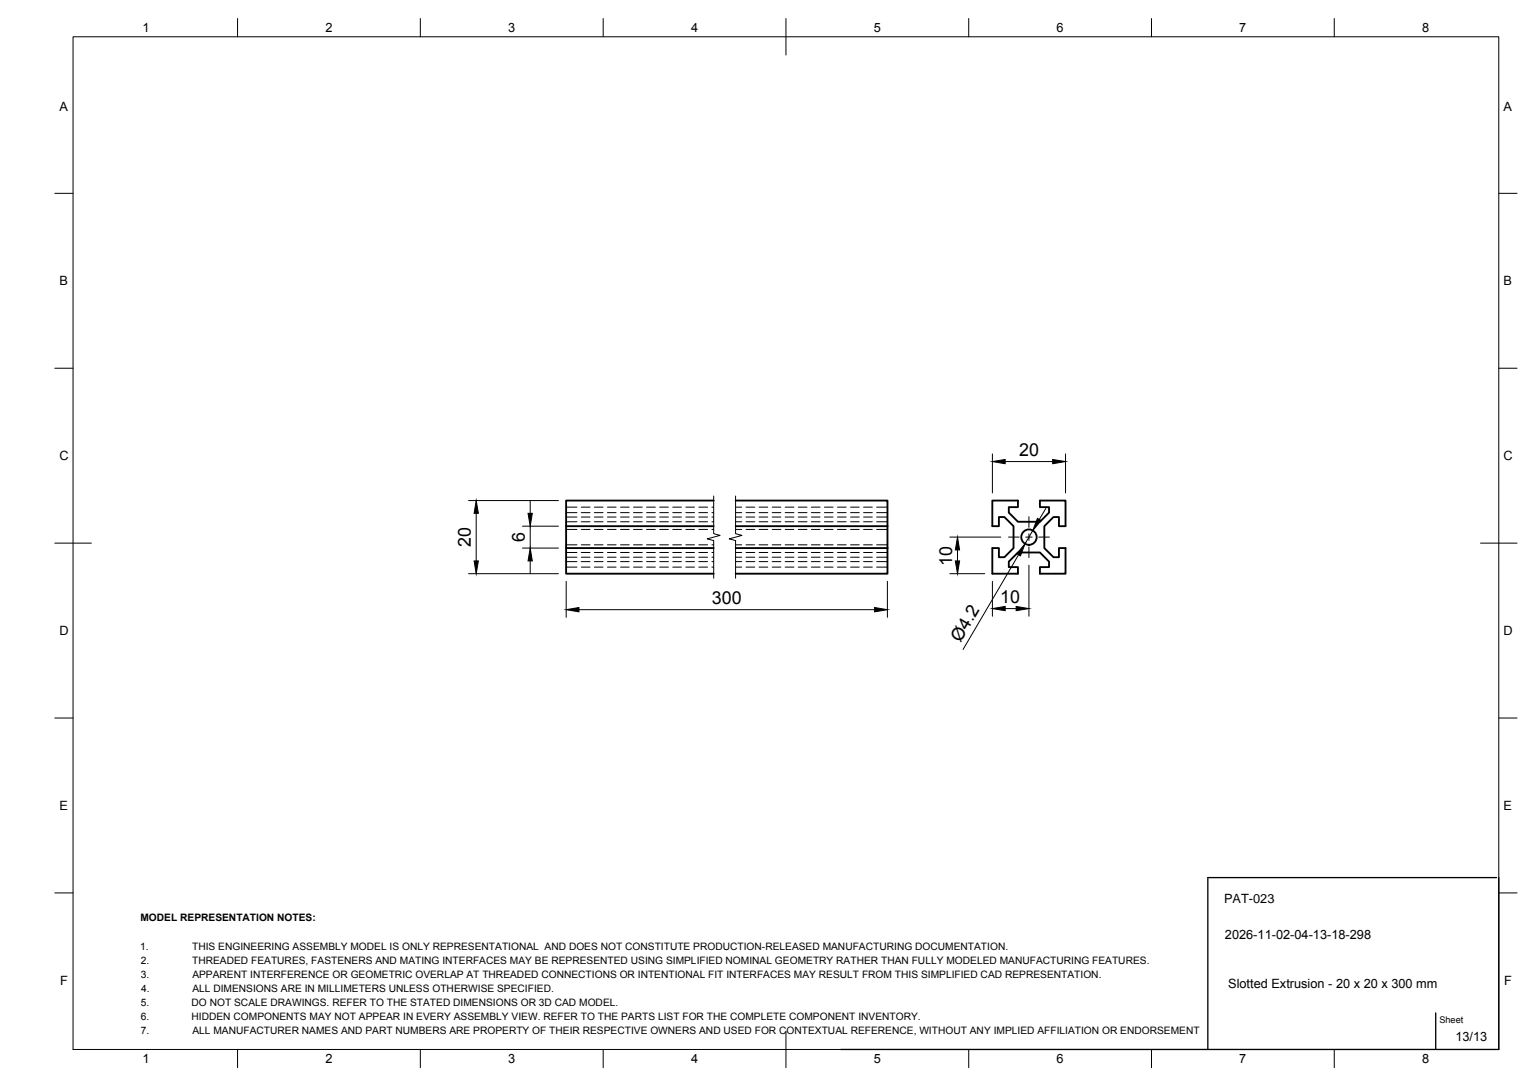
ISO-10303-21;
HEADER;
/* Generated by software containing ST-Developer
 * from STEP Tools, Inc. (www.steptools.com) 
 */

FILE_DESCRIPTION(
/* description */ ('PAT-023'),
/* implementation_level */ '2;1');

FILE_NAME(
/* name */ 'Slotted Extrusion - 20 x 20 x 300 mm.step',
/* time_stamp */ '2026-10-29T15:47:46-07:00',
/* author */ (''),
/* organization */ (''),
/* preprocessor_version */ 'ST-DEVELOPER v20.2',
/* originating_system */ 'Autodesk Translation Framework v15.17.0.0',
/* authorisation */ '');

FILE_SCHEMA (('AUTOMOTIVE_DESIGN { 1 0 10303 214 3 1 1 }'));
ENDSEC;

DATA;
#10=MECHANICAL_DESIGN_GEOMETRIC_PRESENTATION_REPRESENTATION('',(#91),#3773);
#75=SHAPE_REPRESENTATION_RELATIONSHIP('SRR','None',#3824,#83);
#83=ADVANCED_BREP_SHAPE_REPRESENTATION('',(#99),#3772);
#91=STYLED_ITEM('',(#3960),#99);
#99=MANIFOLD_SOLID_BREP('Body1',#2244);
#113=FACE_BOUND('',#468,.T.);
#114=FACE_BOUND('',#470,.T.);
#172=PLANE('',#2450);
#173=PLANE('',#2451);
#174=PLANE('',#2452);
#175=PLANE('',#2453);
#176=PLANE('',#2454);
#177=PLANE('',#2455);
#178=PLANE('',#2456);
#179=PLANE('',#2457);
#180=PLANE('',#2458);
#181=PLANE('',#2459);
#182=PLANE('',#2460);
#183=PLANE('',#2461);
#184=PLANE('',#2462);
#185=PLANE('',#2463);
#186=PLANE('',#2464);
#187=PLANE('',#2465);
#188=PLANE('',#2466);
#189=PLANE('',#2467);
#190=PLANE('',#2468);
#191=PLANE('',#2469);
#192=PLANE('',#2470);
#193=PLANE('',#2471);
#194=PLANE('',#2472);
#195=PLANE('',#2473);
#196=PLANE('',#2474);
#197=PLANE('',#2475);
#198=PLANE('',#2476);
#199=PLANE('',#2477);
#200=PLANE('',#2478);
#201=PLANE('',#2479);
#202=PLANE('',#2480);
#203=PLANE('',#2481);
#204=PLANE('',#2482);
#205=PLANE('',#2483);
#206=PLANE('',#2484);
#207=PLANE('',#2485);
#208=PLANE('',#2489);
#209=PLANE('',#2490);
#210=PLANE('',#2491);
#211=PLANE('',#2492);
#212=PLANE('',#2493);
#213=PLANE('',#2494);
#214=PLANE('',#2495);
#215=PLANE('',#2496);
#216=PLANE('',#2497);
#217=PLANE('',#2498);
#290=FACE_OUTER_BOUND('',#422,.T.);
#291=FACE_OUTER_BOUND('',#423,.T.);
#292=FACE_OUTER_BOUND('',#424,.T.);
#293=FACE_OUTER_BOUND('',#425,.T.);
#294=FACE_OUTER_BOUND('',#426,.T.);
#295=FACE_OUTER_BOUND('',#427,.T.);
#296=FACE_OUTER_BOUND('',#428,.T.);
#297=FACE_OUTER_BOUND('',#429,.T.);
#298=FACE_OUTER_BOUND('',#430,.T.);
#299=FACE_OUTER_BOUND('',#431,.T.);
#300=FACE_OUTER_BOUND('',#432,.T.);
#301=FACE_OUTER_BOUND('',#433,.T.);
#302=FACE_OUTER_BOUND('',#434,.T.);
#303=FACE_OUTER_BOUND('',#435,.T.);
#304=FACE_OUTER_BOUND('',#436,.T.);
#305=FACE_OUTER_BOUND('',#437,.T.);
#306=FACE_OUTER_BOUND('',#438,.T.);
#307=FACE_OUTER_BOUND('',#439,.T.);
#308=FACE_OUTER_BOUND('',#440,.T.);
#309=FACE_OUTER_BOUND('',#441,.T.);
#310=FACE_OUTER_BOUND('',#442,.T.);
#311=FACE_OUTER_BOUND('',#443,.T.);
#312=FACE_OUTER_BOUND('',#444,.T.);
#313=FACE_OUTER_BOUND('',#445,.T.);
#314=FACE_OUTER_BOUND('',#446,.T.);
#315=FACE_OUTER_BOUND('',#447,.T.);
#316=FACE_OUTER_BOUND('',#448,.T.);
#317=FACE_OUTER_BOUND('',#449,.T.);
#318=FACE_OUTER_BOUND('',#450,.T.);
#319=FACE_OUTER_BOUND('',#451,.T.);
#320=FACE_OUTER_BOUND('',#452,.T.);
#321=FACE_OUTER_BOUND('',#453,.T.);
#322=FACE_OUTER_BOUND('',#454,.T.);
#323=FACE_OUTER_BOUND('',#455,.T.);
#324=FACE_OUTER_BOUND('',#456,.T.);
#325=FACE_OUTER_BOUND('',#457,.T.);
#326=FACE_OUTER_BOUND('',#458,.T.);
#327=FACE_OUTER_BOUND('',#459,.T.);
#328=FACE_OUTER_BOUND('',#460,.T.);
#329=FACE_OUTER_BOUND('',#461,.T.);
#330=FACE_OUTER_BOUND('',#462,.T.);
#331=FACE_OUTER_BOUND('',#463,.T.);
#332=FACE_OUTER_BOUND('',#464,.T.);
#333=FACE_OUTER_BOUND('',#465,.T.);
#334=FACE_OUTER_BOUND('',#466,.T.);
#335=FACE_OUTER_BOUND('',#467,.T.);
#336=FACE_OUTER_BOUND('',#469,.T.);
#422=EDGE_LOOP('',(#1839,#1840,#1841,#1842));
#423=EDGE_LOOP('',(#1843,#1844,#1845,#1846));
#424=EDGE_LOOP('',(#1847,#1848,#1849,#1850));
#425=EDGE_LOOP('',(#1851,#1852,#1853,#1854));
#426=EDGE_LOOP('',(#1855,#1856,#1857,#1858));
#427=EDGE_LOOP('',(#1859,#1860,#1861,#1862));
#428=EDGE_LOOP('',(#1863,#1864,#1865,#1866));
#429=EDGE_LOOP('',(#1867,#1868,#1869,#1870));
#430=EDGE_LOOP('',(#1871,#1872,#1873,#1874));
#431=EDGE_LOOP('',(#1875,#1876,#1877,#1878));
#432=EDGE_LOOP('',(#1879,#1880,#1881,#1882));
#433=EDGE_LOOP('',(#1883,#1884,#1885,#1886));
#434=EDGE_LOOP('',(#1887,#1888,#1889,#1890));
#435=EDGE_LOOP('',(#1891,#1892,#1893,#1894));
#436=EDGE_LOOP('',(#1895,#1896,#1897,#1898));
#437=EDGE_LOOP('',(#1899,#1900,#1901,#1902));
#438=EDGE_LOOP('',(#1903,#1904,#1905,#1906));
#439=EDGE_LOOP('',(#1907,#1908,#1909,#1910));
#440=EDGE_LOOP('',(#1911,#1912,#1913,#1914));
#441=EDGE_LOOP('',(#1915,#1916,#1917,#1918));
#442=EDGE_LOOP('',(#1919,#1920,#1921,#1922));
#443=EDGE_LOOP('',(#1923,#1924,#1925,#1926));
#444=EDGE_LOOP('',(#1927,#1928,#1929,#1930));
#445=EDGE_LOOP('',(#1931,#1932,#1933,#1934));
#446=EDGE_LOOP('',(#1935,#1936,#1937,#1938));
#447=EDGE_LOOP('',(#1939,#1940,#1941,#1942));
#448=EDGE_LOOP('',(#1943,#1944,#1945,#1946));
#449=EDGE_LOOP('',(#1947,#1948,#1949,#1950));
#450=EDGE_LOOP('',(#1951,#1952,#1953,#1954));
#451=EDGE_LOOP('',(#1955,#1956,#1957,#1958));
#452=EDGE_LOOP('',(#1959,#1960,#1961,#1962));
#453=EDGE_LOOP('',(#1963,#1964,#1965,#1966));
#454=EDGE_LOOP('',(#1967,#1968,#1969,#1970));
#455=EDGE_LOOP('',(#1971,#1972,#1973,#1974));
#456=EDGE_LOOP('',(#1975,#1976,#1977,#1978));
#457=EDGE_LOOP('',(#1979,#1980,#1981,#1982));
#458=EDGE_LOOP('',(#1983,#1984,#1985,#1986));
#459=EDGE_LOOP('',(#1987,#1988,#1989,#1990));
#460=EDGE_LOOP('',(#1991,#1992,#1993,#1994));
#461=EDGE_LOOP('',(#1995,#1996,#1997,#1998));
#462=EDGE_LOOP('',(#1999,#2000,#2001,#2002));
#463=EDGE_LOOP('',(#2003,#2004,#2005,#2006));
#464=EDGE_LOOP('',(#2007,#2008,#2009,#2010));
#465=EDGE_LOOP('',(#2011,#2012,#2013,#2014));
#466=EDGE_LOOP('',(#2015,#2016,#2017,#2018));
#467=EDGE_LOOP('',(#2019,#2020,#2021,#2022,#2023,#2024,#2025,#2026,#2027,
#2028,#2029,#2030,#2031,#2032,#2033,#2034,#2035,#2036,#2037,#2038,#2039,
#2040,#2041,#2042,#2043,#2044,#2045,#2046,#2047,#2048,#2049,#2050,#2051,
#2052,#2053,#2054,#2055,#2056,#2057,#2058,#2059,#2060,#2061,#2062));
#468=EDGE_LOOP('',(#2063));
#469=EDGE_LOOP('',(#2064,#2065,#2066,#2067,#2068,#2069,#2070,#2071,#2072,
#2073,#2074,#2075,#2076,#2077,#2078,#2079,#2080,#2081,#2082,#2083,#2084,
#2085,#2086,#2087,#2088,#2089,#2090,#2091,#2092,#2093,#2094,#2095,#2096,
#2097,#2098,#2099,#2100,#2101,#2102,#2103,#2104,#2105,#2106,#2107));
#470=EDGE_LOOP('',(#2108));
#602=LINE('',#3476,#866);
#603=LINE('',#3478,#867);
#604=LINE('',#3480,#868);
#605=LINE('',#3481,#869);
#606=LINE('',#3484,#870);
#607=LINE('',#3486,#871);
#608=LINE('',#3487,#872);
#609=LINE('',#3490,#873);
#610=LINE('',#3492,#874);
#611=LINE('',#3493,#875);
#612=LINE('',#3496,#876);
#613=LINE('',#3498,#877);
#614=LINE('',#3499,#878);
#615=LINE('',#3502,#879);
#616=LINE('',#3504,#880);
#617=LINE('',#3505,#881);
#618=LINE('',#3508,#882);
#619=LINE('',#3510,#883);
#620=LINE('',#3511,#884);
#621=LINE('',#3514,#885);
#622=LINE('',#3516,#886);
#623=LINE('',#3517,#887);
#624=LINE('',#3520,#888);
#625=LINE('',#3522,#889);
#626=LINE('',#3523,#890);
#627=LINE('',#3526,#891);
#628=LINE('',#3528,#892);
#629=LINE('',#3529,#893);
#630=LINE('',#3533,#894);
#631=LINE('',#3535,#895);
#632=LINE('',#3537,#896);
#633=LINE('',#3538,#897);
#634=LINE('',#3541,#898);
#635=LINE('',#3543,#899);
#636=LINE('',#3544,#900);
#637=LINE('',#3547,#901);
#638=LINE('',#3549,#902);
#639=LINE('',#3550,#903);
#640=LINE('',#3553,#904);
#641=LINE('',#3555,#905);
#642=LINE('',#3556,#906);
#643=LINE('',#3559,#907);
#644=LINE('',#3561,#908);
#645=LINE('',#3562,#909);
#646=LINE('',#3565,#910);
#647=LINE('',#3567,#911);
#648=LINE('',#3568,#912);
#649=LINE('',#3571,#913);
#650=LINE('',#3573,#914);
#651=LINE('',#3574,#915);
#652=LINE('',#3577,#916);
#653=LINE('',#3579,#917);
#654=LINE('',#3580,#918);
#655=LINE('',#3583,#919);
#656=LINE('',#3585,#920);
#657=LINE('',#3586,#921);
#658=LINE('',#3590,#922);
#659=LINE('',#3592,#923);
#660=LINE('',#3594,#924);
#661=LINE('',#3595,#925);
#662=LINE('',#3598,#926);
#663=LINE('',#3600,#927);
#664=LINE('',#3601,#928);
#665=LINE('',#3604,#929);
#666=LINE('',#3606,#930);
#667=LINE('',#3607,#931);
#668=LINE('',#3610,#932);
#669=LINE('',#3612,#933);
#670=LINE('',#3613,#934);
#671=LINE('',#3616,#935);
#672=LINE('',#3618,#936);
#673=LINE('',#3619,#937);
#674=LINE('',#3622,#938);
#675=LINE('',#3624,#939);
#676=LINE('',#3625,#940);
#677=LINE('',#3628,#941);
#678=LINE('',#3630,#942);
#679=LINE('',#3631,#943);
#680=LINE('',#3634,#944);
#681=LINE('',#3636,#945);
#682=LINE('',#3637,#946);
#683=LINE('',#3640,#947);
#684=LINE('',#3642,#948);
#685=LINE('',#3643,#949);
#686=LINE('',#3647,#950);
#687=LINE('',#3649,#951);
#688=LINE('',#3651,#952);
#689=LINE('',#3652,#953);
#690=LINE('',#3655,#954);
#691=LINE('',#3657,#955);
#692=LINE('',#3658,#956);
#693=LINE('',#3661,#957);
#694=LINE('',#3663,#958);
#695=LINE('',#3664,#959);
#696=LINE('',#3667,#960);
#697=LINE('',#3669,#961);
#698=LINE('',#3670,#962);
#699=LINE('',#3673,#963);
#700=LINE('',#3675,#964);
#701=LINE('',#3676,#965);
#702=LINE('',#3679,#966);
#703=LINE('',#3681,#967);
#704=LINE('',#3682,#968);
#705=LINE('',#3685,#969);
#706=LINE('',#3687,#970);
#707=LINE('',#3688,#971);
#708=LINE('',#3691,#972);
#709=LINE('',#3693,#973);
#710=LINE('',#3694,#974);
#711=LINE('',#3697,#975);
#712=LINE('',#3699,#976);
#713=LINE('',#3700,#977);
#714=LINE('',#3705,#978);
#715=LINE('',#3709,#979);
#716=LINE('',#3711,#980);
#717=LINE('',#3712,#981);
#718=LINE('',#3715,#982);
#719=LINE('',#3717,#983);
#720=LINE('',#3718,#984);
#721=LINE('',#3720,#985);
#722=LINE('',#3721,#986);
#723=LINE('',#3724,#987);
#724=LINE('',#3726,#988);
#725=LINE('',#3727,#989);
#726=LINE('',#3729,#990);
#727=LINE('',#3730,#991);
#728=LINE('',#3733,#992);
#729=LINE('',#3735,#993);
#730=LINE('',#3736,#994);
#731=LINE('',#3738,#995);
#732=LINE('',#3739,#996);
#733=LINE('',#3741,#997);
#734=LINE('',#3742,#998);
#866=VECTOR('',#2867,1.);
#867=VECTOR('',#2868,1.);
#868=VECTOR('',#2869,1.);
#869=VECTOR('',#2870,1.);
#870=VECTOR('',#2873,1.);
#871=VECTOR('',#2874,1.);
#872=VECTOR('',#2875,1.);
#873=VECTOR('',#2878,1.);
#874=VECTOR('',#2879,1.);
#875=VECTOR('',#2880,1.);
#876=VECTOR('',#2883,1.);
#877=VECTOR('',#2884,1.);
#878=VECTOR('',#2885,1.);
#879=VECTOR('',#2888,1.);
#880=VECTOR('',#2889,1.);
#881=VECTOR('',#2890,1.);
#882=VECTOR('',#2893,1.);
#883=VECTOR('',#2894,1.);
#884=VECTOR('',#2895,1.);
#885=VECTOR('',#2898,1.);
#886=VECTOR('',#2899,1.);
#887=VECTOR('',#2900,1.);
#888=VECTOR('',#2903,1.);
#889=VECTOR('',#2904,1.);
#890=VECTOR('',#2905,1.);
#891=VECTOR('',#2908,1.);
#892=VECTOR('',#2909,1.);
#893=VECTOR('',#2910,1.);
#894=VECTOR('',#2913,1.);
#895=VECTOR('',#2914,1.);
#896=VECTOR('',#2915,1.);
#897=VECTOR('',#2916,1.);
#898=VECTOR('',#2919,1.);
#899=VECTOR('',#2920,1.);
#900=VECTOR('',#2921,1.);
#901=VECTOR('',#2924,1.);
#902=VECTOR('',#2925,1.);
#903=VECTOR('',#2926,1.);
#904=VECTOR('',#2929,1.);
#905=VECTOR('',#2930,1.);
#906=VECTOR('',#2931,1.);
#907=VECTOR('',#2934,1.);
#908=VECTOR('',#2935,1.);
#909=VECTOR('',#2936,1.);
#910=VECTOR('',#2939,1.);
#911=VECTOR('',#2940,1.);
#912=VECTOR('',#2941,1.);
#913=VECTOR('',#2944,1.);
#914=VECTOR('',#2945,1.);
#915=VECTOR('',#2946,1.);
#916=VECTOR('',#2949,1.);
#917=VECTOR('',#2950,1.);
#918=VECTOR('',#2951,1.);
#919=VECTOR('',#2954,1.);
#920=VECTOR('',#2955,1.);
#921=VECTOR('',#2956,1.);
#922=VECTOR('',#2959,1.);
#923=VECTOR('',#2960,1.);
#924=VECTOR('',#2961,1.);
#925=VECTOR('',#2962,1.);
#926=VECTOR('',#2965,1.);
#927=VECTOR('',#2966,1.);
#928=VECTOR('',#2967,1.);
#929=VECTOR('',#2970,1.);
#930=VECTOR('',#2971,1.);
#931=VECTOR('',#2972,1.);
#932=VECTOR('',#2975,1.);
#933=VECTOR('',#2976,1.);
#934=VECTOR('',#2977,1.);
#935=VECTOR('',#2980,1.);
#936=VECTOR('',#2981,1.);
#937=VECTOR('',#2982,1.);
#938=VECTOR('',#2985,1.);
#939=VECTOR('',#2986,1.);
#940=VECTOR('',#2987,1.);
#941=VECTOR('',#2990,1.);
#942=VECTOR('',#2991,1.);
#943=VECTOR('',#2992,1.);
#944=VECTOR('',#2995,1.);
#945=VECTOR('',#2996,1.);
#946=VECTOR('',#2997,1.);
#947=VECTOR('',#3000,1.);
#948=VECTOR('',#3001,1.);
#949=VECTOR('',#3002,1.);
#950=VECTOR('',#3005,1.);
#951=VECTOR('',#3006,1.);
#952=VECTOR('',#3007,1.);
#953=VECTOR('',#3008,1.);
#954=VECTOR('',#3011,1.);
#955=VECTOR('',#3012,1.);
#956=VECTOR('',#3013,1.);
#957=VECTOR('',#3016,1.);
#958=VECTOR('',#3017,1.);
#959=VECTOR('',#3018,1.);
#960=VECTOR('',#3021,1.);
#961=VECTOR('',#3022,1.);
#962=VECTOR('',#3023,1.);
#963=VECTOR('',#3026,1.);
#964=VECTOR('',#3027,1.);
#965=VECTOR('',#3028,1.);
#966=VECTOR('',#3031,1.);
#967=VECTOR('',#3032,1.);
#968=VECTOR('',#3033,1.);
#969=VECTOR('',#3036,1.);
#970=VECTOR('',#3037,1.);
#971=VECTOR('',#3038,1.);
#972=VECTOR('',#3041,1.);
#973=VECTOR('',#3042,1.);
#974=VECTOR('',#3043,1.);
#975=VECTOR('',#3046,1.);
#976=VECTOR('',#3047,1.);
#977=VECTOR('',#3048,1.);
#978=VECTOR('',#3053,0.21);
#979=VECTOR('',#3058,1.);
#980=VECTOR('',#3059,1.);
#981=VECTOR('',#3060,1.);
#982=VECTOR('',#3063,1.);
#983=VECTOR('',#3064,1.);
#984=VECTOR('',#3065,1.);
#985=VECTOR('',#3068,1.);
#986=VECTOR('',#3069,1.);
#987=VECTOR('',#3072,1.);
#988=VECTOR('',#3073,1.);
#989=VECTOR('',#3074,1.);
#990=VECTOR('',#3077,1.);
#991=VECTOR('',#3078,1.);
#992=VECTOR('',#3081,1.);
#993=VECTOR('',#3082,1.);
#994=VECTOR('',#3083,1.);
#995=VECTOR('',#3086,1.);
#996=VECTOR('',#3087,1.);
#997=VECTOR('',#3090,1.);
#998=VECTOR('',#3091,1.);
#1023=CIRCLE('',#2487,0.21);
#1024=CIRCLE('',#2488,0.21);
#1131=VERTEX_POINT('',#3474);
#1132=VERTEX_POINT('',#3475);
#1133=VERTEX_POINT('',#3477);
#1134=VERTEX_POINT('',#3479);
#1135=VERTEX_POINT('',#3483);
#1136=VERTEX_POINT('',#3485);
#1137=VERTEX_POINT('',#3489);
#1138=VERTEX_POINT('',#3491);
#1139=VERTEX_POINT('',#3495);
#1140=VERTEX_POINT('',#3497);
#1141=VERTEX_POINT('',#3501);
#1142=VERTEX_POINT('',#3503);
#1143=VERTEX_POINT('',#3507);
#1144=VERTEX_POINT('',#3509);
#1145=VERTEX_POINT('',#3513);
#1146=VERTEX_POINT('',#3515);
#1147=VERTEX_POINT('',#3519);
#1148=VERTEX_POINT('',#3521);
#1149=VERTEX_POINT('',#3525);
#1150=VERTEX_POINT('',#3527);
#1151=VERTEX_POINT('',#3531);
#1152=VERTEX_POINT('',#3532);
#1153=VERTEX_POINT('',#3534);
#1154=VERTEX_POINT('',#3536);
#1155=VERTEX_POINT('',#3540);
#1156=VERTEX_POINT('',#3542);
#1157=VERTEX_POINT('',#3546);
#1158=VERTEX_POINT('',#3548);
#1159=VERTEX_POINT('',#3552);
#1160=VERTEX_POINT('',#3554);
#1161=VERTEX_POINT('',#3558);
#1162=VERTEX_POINT('',#3560);
#1163=VERTEX_POINT('',#3564);
#1164=VERTEX_POINT('',#3566);
#1165=VERTEX_POINT('',#3570);
#1166=VERTEX_POINT('',#3572);
#1167=VERTEX_POINT('',#3576);
#1168=VERTEX_POINT('',#3578);
#1169=VERTEX_POINT('',#3582);
#1170=VERTEX_POINT('',#3584);
#1171=VERTEX_POINT('',#3588);
#1172=VERTEX_POINT('',#3589);
#1173=VERTEX_POINT('',#3591);
#1174=VERTEX_POINT('',#3593);
#1175=VERTEX_POINT('',#3597);
#1176=VERTEX_POINT('',#3599);
#1177=VERTEX_POINT('',#3603);
#1178=VERTEX_POINT('',#3605);
#1179=VERTEX_POINT('',#3609);
#1180=VERTEX_POINT('',#3611);
#1181=VERTEX_POINT('',#3615);
#1182=VERTEX_POINT('',#3617);
#1183=VERTEX_POINT('',#3621);
#1184=VERTEX_POINT('',#3623);
#1185=VERTEX_POINT('',#3627);
#1186=VERTEX_POINT('',#3629);
#1187=VERTEX_POINT('',#3633);
#1188=VERTEX_POINT('',#3635);
#1189=VERTEX_POINT('',#3639);
#1190=VERTEX_POINT('',#3641);
#1191=VERTEX_POINT('',#3645);
#1192=VERTEX_POINT('',#3646);
#1193=VERTEX_POINT('',#3648);
#1194=VERTEX_POINT('',#3650);
#1195=VERTEX_POINT('',#3654);
#1196=VERTEX_POINT('',#3656);
#1197=VERTEX_POINT('',#3660);
#1198=VERTEX_POINT('',#3662);
#1199=VERTEX_POINT('',#3666);
#1200=VERTEX_POINT('',#3668);
#1201=VERTEX_POINT('',#3672);
#1202=VERTEX_POINT('',#3674);
#1203=VERTEX_POINT('',#3678);
#1204=VERTEX_POINT('',#3680);
#1205=VERTEX_POINT('',#3684);
#1206=VERTEX_POINT('',#3686);
#1207=VERTEX_POINT('',#3690);
#1208=VERTEX_POINT('',#3692);
#1209=VERTEX_POINT('',#3696);
#1210=VERTEX_POINT('',#3698);
#1211=VERTEX_POINT('',#3702);
#1212=VERTEX_POINT('',#3704);
#1213=VERTEX_POINT('',#3708);
#1214=VERTEX_POINT('',#3710);
#1215=VERTEX_POINT('',#3714);
#1216=VERTEX_POINT('',#3716);
#1217=VERTEX_POINT('',#3723);
#1218=VERTEX_POINT('',#3725);
#1219=VERTEX_POINT('',#3732);
#1220=VERTEX_POINT('',#3734);
#1382=EDGE_CURVE('',#1131,#1132,#602,.T.);
#1383=EDGE_CURVE('',#1131,#1133,#603,.T.);
#1384=EDGE_CURVE('',#1134,#1133,#604,.T.);
#1385=EDGE_CURVE('',#1132,#1134,#605,.T.);
#1386=EDGE_CURVE('',#1135,#1131,#606,.T.);
#1387=EDGE_CURVE('',#1135,#1136,#607,.T.);
#1388=EDGE_CURVE('',#1133,#1136,#608,.T.);
#1389=EDGE_CURVE('',#1137,#1135,#609,.T.);
#1390=EDGE_CURVE('',#1137,#1138,#610,.T.);
#1391=EDGE_CURVE('',#1136,#1138,#611,.T.);
#1392=EDGE_CURVE('',#1139,#1137,#612,.T.);
#1393=EDGE_CURVE('',#1139,#1140,#613,.T.);
#1394=EDGE_CURVE('',#1138,#1140,#614,.T.);
#1395=EDGE_CURVE('',#1141,#1139,#615,.T.);
#1396=EDGE_CURVE('',#1141,#1142,#616,.T.);
#1397=EDGE_CURVE('',#1140,#1142,#617,.T.);
#1398=EDGE_CURVE('',#1143,#1141,#618,.T.);
#1399=EDGE_CURVE('',#1143,#1144,#619,.T.);
#1400=EDGE_CURVE('',#1142,#1144,#620,.T.);
#1401=EDGE_CURVE('',#1145,#1143,#621,.T.);
#1402=EDGE_CURVE('',#1145,#1146,#622,.T.);
#1403=EDGE_CURVE('',#1144,#1146,#623,.T.);
#1404=EDGE_CURVE('',#1147,#1145,#624,.T.);
#1405=EDGE_CURVE('',#1147,#1148,#625,.T.);
#1406=EDGE_CURVE('',#1146,#1148,#626,.T.);
#1407=EDGE_CURVE('',#1149,#1147,#627,.T.);
#1408=EDGE_CURVE('',#1150,#1149,#628,.T.);
#1409=EDGE_CURVE('',#1148,#1150,#629,.T.);
#1410=EDGE_CURVE('',#1151,#1152,#630,.T.);
#1411=EDGE_CURVE('',#1151,#1153,#631,.T.);
#1412=EDGE_CURVE('',#1154,#1153,#632,.T.);
#1413=EDGE_CURVE('',#1152,#1154,#633,.T.);
#1414=EDGE_CURVE('',#1155,#1151,#634,.T.);
#1415=EDGE_CURVE('',#1155,#1156,#635,.T.);
#1416=EDGE_CURVE('',#1153,#1156,#636,.T.);
#1417=EDGE_CURVE('',#1157,#1155,#637,.T.);
#1418=EDGE_CURVE('',#1157,#1158,#638,.T.);
#1419=EDGE_CURVE('',#1156,#1158,#639,.T.);
#1420=EDGE_CURVE('',#1159,#1157,#640,.T.);
#1421=EDGE_CURVE('',#1159,#1160,#641,.T.);
#1422=EDGE_CURVE('',#1158,#1160,#642,.T.);
#1423=EDGE_CURVE('',#1161,#1159,#643,.T.);
#1424=EDGE_CURVE('',#1161,#1162,#644,.T.);
#1425=EDGE_CURVE('',#1160,#1162,#645,.T.);
#1426=EDGE_CURVE('',#1163,#1161,#646,.T.);
#1427=EDGE_CURVE('',#1163,#1164,#647,.T.);
#1428=EDGE_CURVE('',#1162,#1164,#648,.T.);
#1429=EDGE_CURVE('',#1165,#1163,#649,.T.);
#1430=EDGE_CURVE('',#1165,#1166,#650,.T.);
#1431=EDGE_CURVE('',#1164,#1166,#651,.T.);
#1432=EDGE_CURVE('',#1167,#1165,#652,.T.);
#1433=EDGE_CURVE('',#1167,#1168,#653,.T.);
#1434=EDGE_CURVE('',#1166,#1168,#654,.T.);
#1435=EDGE_CURVE('',#1169,#1167,#655,.T.);
#1436=EDGE_CURVE('',#1170,#1169,#656,.T.);
#1437=EDGE_CURVE('',#1168,#1170,#657,.T.);
#1438=EDGE_CURVE('',#1171,#1172,#658,.T.);
#1439=EDGE_CURVE('',#1171,#1173,#659,.T.);
#1440=EDGE_CURVE('',#1174,#1173,#660,.T.);
#1441=EDGE_CURVE('',#1172,#1174,#661,.T.);
#1442=EDGE_CURVE('',#1175,#1171,#662,.T.);
#1443=EDGE_CURVE('',#1175,#1176,#663,.T.);
#1444=EDGE_CURVE('',#1173,#1176,#664,.T.);
#1445=EDGE_CURVE('',#1177,#1175,#665,.T.);
#1446=EDGE_CURVE('',#1177,#1178,#666,.T.);
#1447=EDGE_CURVE('',#1176,#1178,#667,.T.);
#1448=EDGE_CURVE('',#1179,#1177,#668,.T.);
#1449=EDGE_CURVE('',#1179,#1180,#669,.T.);
#1450=EDGE_CURVE('',#1178,#1180,#670,.T.);
#1451=EDGE_CURVE('',#1181,#1179,#671,.T.);
#1452=EDGE_CURVE('',#1181,#1182,#672,.T.);
#1453=EDGE_CURVE('',#1180,#1182,#673,.T.);
#1454=EDGE_CURVE('',#1183,#1181,#674,.T.);
#1455=EDGE_CURVE('',#1183,#1184,#675,.T.);
#1456=EDGE_CURVE('',#1182,#1184,#676,.T.);
#1457=EDGE_CURVE('',#1185,#1183,#677,.T.);
#1458=EDGE_CURVE('',#1185,#1186,#678,.T.);
#1459=EDGE_CURVE('',#1184,#1186,#679,.T.);
#1460=EDGE_CURVE('',#1187,#1185,#680,.T.);
#1461=EDGE_CURVE('',#1187,#1188,#681,.T.);
#1462=EDGE_CURVE('',#1186,#1188,#682,.T.);
#1463=EDGE_CURVE('',#1189,#1187,#683,.T.);
#1464=EDGE_CURVE('',#1190,#1189,#684,.T.);
#1465=EDGE_CURVE('',#1188,#1190,#685,.T.);
#1466=EDGE_CURVE('',#1191,#1192,#686,.T.);
#1467=EDGE_CURVE('',#1191,#1193,#687,.T.);
#1468=EDGE_CURVE('',#1194,#1193,#688,.T.);
#1469=EDGE_CURVE('',#1192,#1194,#689,.T.);
#1470=EDGE_CURVE('',#1195,#1191,#690,.T.);
#1471=EDGE_CURVE('',#1195,#1196,#691,.T.);
#1472=EDGE_CURVE('',#1193,#1196,#692,.T.);
#1473=EDGE_CURVE('',#1197,#1195,#693,.T.);
#1474=EDGE_CURVE('',#1197,#1198,#694,.T.);
#1475=EDGE_CURVE('',#1196,#1198,#695,.T.);
#1476=EDGE_CURVE('',#1199,#1197,#696,.T.);
#1477=EDGE_CURVE('',#1199,#1200,#697,.T.);
#1478=EDGE_CURVE('',#1198,#1200,#698,.T.);
#1479=EDGE_CURVE('',#1201,#1199,#699,.T.);
#1480=EDGE_CURVE('',#1201,#1202,#700,.T.);
#1481=EDGE_CURVE('',#1200,#1202,#701,.T.);
#1482=EDGE_CURVE('',#1203,#1201,#702,.T.);
#1483=EDGE_CURVE('',#1203,#1204,#703,.T.);
#1484=EDGE_CURVE('',#1202,#1204,#704,.T.);
#1485=EDGE_CURVE('',#1205,#1203,#705,.T.);
#1486=EDGE_CURVE('',#1205,#1206,#706,.T.);
#1487=EDGE_CURVE('',#1204,#1206,#707,.T.);
#1488=EDGE_CURVE('',#1207,#1205,#708,.T.);
#1489=EDGE_CURVE('',#1207,#1208,#709,.T.);
#1490=EDGE_CURVE('',#1206,#1208,#710,.T.);
#1491=EDGE_CURVE('',#1209,#1207,#711,.T.);
#1492=EDGE_CURVE('',#1210,#1209,#712,.T.);
#1493=EDGE_CURVE('',#1208,#1210,#713,.T.);
#1494=EDGE_CURVE('',#1211,#1211,#1023,.T.);
#1495=EDGE_CURVE('',#1211,#1212,#714,.T.);
#1496=EDGE_CURVE('',#1212,#1212,#1024,.T.);
#1497=EDGE_CURVE('',#1149,#1213,#715,.T.);
#1498=EDGE_CURVE('',#1213,#1214,#716,.T.);
#1499=EDGE_CURVE('',#1150,#1214,#717,.T.);
#1500=EDGE_CURVE('',#1215,#1134,#718,.T.);
#1501=EDGE_CURVE('',#1216,#1215,#719,.T.);
#1502=EDGE_CURVE('',#1216,#1132,#720,.T.);
#1503=EDGE_CURVE('',#1169,#1216,#721,.T.);
#1504=EDGE_CURVE('',#1170,#1215,#722,.T.);
#1505=EDGE_CURVE('',#1217,#1154,#723,.T.);
#1506=EDGE_CURVE('',#1218,#1217,#724,.T.);
#1507=EDGE_CURVE('',#1218,#1152,#725,.T.);
#1508=EDGE_CURVE('',#1189,#1218,#726,.T.);
#1509=EDGE_CURVE('',#1190,#1217,#727,.T.);
#1510=EDGE_CURVE('',#1219,#1174,#728,.T.);
#1511=EDGE_CURVE('',#1220,#1219,#729,.T.);
#1512=EDGE_CURVE('',#1220,#1172,#730,.T.);
#1513=EDGE_CURVE('',#1209,#1220,#731,.T.);
#1514=EDGE_CURVE('',#1210,#1219,#732,.T.);
#1515=EDGE_CURVE('',#1214,#1194,#733,.T.);
#1516=EDGE_CURVE('',#1213,#1192,#734,.T.);
#1839=ORIENTED_EDGE('',*,*,#1382,.F.);
#1840=ORIENTED_EDGE('',*,*,#1383,.T.);
#1841=ORIENTED_EDGE('',*,*,#1384,.F.);
#1842=ORIENTED_EDGE('',*,*,#1385,.F.);
#1843=ORIENTED_EDGE('',*,*,#1386,.F.);
#1844=ORIENTED_EDGE('',*,*,#1387,.T.);
#1845=ORIENTED_EDGE('',*,*,#1388,.F.);
#1846=ORIENTED_EDGE('',*,*,#1383,.F.);
#1847=ORIENTED_EDGE('',*,*,#1389,.F.);
#1848=ORIENTED_EDGE('',*,*,#1390,.T.);
#1849=ORIENTED_EDGE('',*,*,#1391,.F.);
#1850=ORIENTED_EDGE('',*,*,#1387,.F.);
#1851=ORIENTED_EDGE('',*,*,#1392,.F.);
#1852=ORIENTED_EDGE('',*,*,#1393,.T.);
#1853=ORIENTED_EDGE('',*,*,#1394,.F.);
#1854=ORIENTED_EDGE('',*,*,#1390,.F.);
#1855=ORIENTED_EDGE('',*,*,#1395,.F.);
#1856=ORIENTED_EDGE('',*,*,#1396,.T.);
#1857=ORIENTED_EDGE('',*,*,#1397,.F.);
#1858=ORIENTED_EDGE('',*,*,#1393,.F.);
#1859=ORIENTED_EDGE('',*,*,#1398,.F.);
#1860=ORIENTED_EDGE('',*,*,#1399,.T.);
#1861=ORIENTED_EDGE('',*,*,#1400,.F.);
#1862=ORIENTED_EDGE('',*,*,#1396,.F.);
#1863=ORIENTED_EDGE('',*,*,#1401,.F.);
#1864=ORIENTED_EDGE('',*,*,#1402,.T.);
#1865=ORIENTED_EDGE('',*,*,#1403,.F.);
#1866=ORIENTED_EDGE('',*,*,#1399,.F.);
#1867=ORIENTED_EDGE('',*,*,#1404,.F.);
#1868=ORIENTED_EDGE('',*,*,#1405,.T.);
#1869=ORIENTED_EDGE('',*,*,#1406,.F.);
#1870=ORIENTED_EDGE('',*,*,#1402,.F.);
#1871=ORIENTED_EDGE('',*,*,#1407,.F.);
#1872=ORIENTED_EDGE('',*,*,#1408,.F.);
#1873=ORIENTED_EDGE('',*,*,#1409,.F.);
#1874=ORIENTED_EDGE('',*,*,#1405,.F.);
#1875=ORIENTED_EDGE('',*,*,#1410,.F.);
#1876=ORIENTED_EDGE('',*,*,#1411,.T.);
#1877=ORIENTED_EDGE('',*,*,#1412,.F.);
#1878=ORIENTED_EDGE('',*,*,#1413,.F.);
#1879=ORIENTED_EDGE('',*,*,#1414,.F.);
#1880=ORIENTED_EDGE('',*,*,#1415,.T.);
#1881=ORIENTED_EDGE('',*,*,#1416,.F.);
#1882=ORIENTED_EDGE('',*,*,#1411,.F.);
#1883=ORIENTED_EDGE('',*,*,#1417,.F.);
#1884=ORIENTED_EDGE('',*,*,#1418,.T.);
#1885=ORIENTED_EDGE('',*,*,#1419,.F.);
#1886=ORIENTED_EDGE('',*,*,#1415,.F.);
#1887=ORIENTED_EDGE('',*,*,#1420,.F.);
#1888=ORIENTED_EDGE('',*,*,#1421,.T.);
#1889=ORIENTED_EDGE('',*,*,#1422,.F.);
#1890=ORIENTED_EDGE('',*,*,#1418,.F.);
#1891=ORIENTED_EDGE('',*,*,#1423,.F.);
#1892=ORIENTED_EDGE('',*,*,#1424,.T.);
#1893=ORIENTED_EDGE('',*,*,#1425,.F.);
#1894=ORIENTED_EDGE('',*,*,#1421,.F.);
#1895=ORIENTED_EDGE('',*,*,#1426,.F.);
#1896=ORIENTED_EDGE('',*,*,#1427,.T.);
#1897=ORIENTED_EDGE('',*,*,#1428,.F.);
#1898=ORIENTED_EDGE('',*,*,#1424,.F.);
#1899=ORIENTED_EDGE('',*,*,#1429,.F.);
#1900=ORIENTED_EDGE('',*,*,#1430,.T.);
#1901=ORIENTED_EDGE('',*,*,#1431,.F.);
#1902=ORIENTED_EDGE('',*,*,#1427,.F.);
#1903=ORIENTED_EDGE('',*,*,#1432,.F.);
#1904=ORIENTED_EDGE('',*,*,#1433,.T.);
#1905=ORIENTED_EDGE('',*,*,#1434,.F.);
#1906=ORIENTED_EDGE('',*,*,#1430,.F.);
#1907=ORIENTED_EDGE('',*,*,#1435,.F.);
#1908=ORIENTED_EDGE('',*,*,#1436,.F.);
#1909=ORIENTED_EDGE('',*,*,#1437,.F.);
#1910=ORIENTED_EDGE('',*,*,#1433,.F.);
#1911=ORIENTED_EDGE('',*,*,#1438,.F.);
#1912=ORIENTED_EDGE('',*,*,#1439,.T.);
#1913=ORIENTED_EDGE('',*,*,#1440,.F.);
#1914=ORIENTED_EDGE('',*,*,#1441,.F.);
#1915=ORIENTED_EDGE('',*,*,#1442,.F.);
#1916=ORIENTED_EDGE('',*,*,#1443,.T.);
#1917=ORIENTED_EDGE('',*,*,#1444,.F.);
#1918=ORIENTED_EDGE('',*,*,#1439,.F.);
#1919=ORIENTED_EDGE('',*,*,#1445,.F.);
#1920=ORIENTED_EDGE('',*,*,#1446,.T.);
#1921=ORIENTED_EDGE('',*,*,#1447,.F.);
#1922=ORIENTED_EDGE('',*,*,#1443,.F.);
#1923=ORIENTED_EDGE('',*,*,#1448,.F.);
#1924=ORIENTED_EDGE('',*,*,#1449,.T.);
#1925=ORIENTED_EDGE('',*,*,#1450,.F.);
#1926=ORIENTED_EDGE('',*,*,#1446,.F.);
#1927=ORIENTED_EDGE('',*,*,#1451,.F.);
#1928=ORIENTED_EDGE('',*,*,#1452,.T.);
#1929=ORIENTED_EDGE('',*,*,#1453,.F.);
#1930=ORIENTED_EDGE('',*,*,#1449,.F.);
#1931=ORIENTED_EDGE('',*,*,#1454,.F.);
#1932=ORIENTED_EDGE('',*,*,#1455,.T.);
#1933=ORIENTED_EDGE('',*,*,#1456,.F.);
#1934=ORIENTED_EDGE('',*,*,#1452,.F.);
#1935=ORIENTED_EDGE('',*,*,#1457,.F.);
#1936=ORIENTED_EDGE('',*,*,#1458,.T.);
#1937=ORIENTED_EDGE('',*,*,#1459,.F.);
#1938=ORIENTED_EDGE('',*,*,#1455,.F.);
#1939=ORIENTED_EDGE('',*,*,#1460,.F.);
#1940=ORIENTED_EDGE('',*,*,#1461,.T.);
#1941=ORIENTED_EDGE('',*,*,#1462,.F.);
#1942=ORIENTED_EDGE('',*,*,#1458,.F.);
#1943=ORIENTED_EDGE('',*,*,#1463,.F.);
#1944=ORIENTED_EDGE('',*,*,#1464,.F.);
#1945=ORIENTED_EDGE('',*,*,#1465,.F.);
#1946=ORIENTED_EDGE('',*,*,#1461,.F.);
#1947=ORIENTED_EDGE('',*,*,#1466,.F.);
#1948=ORIENTED_EDGE('',*,*,#1467,.T.);
#1949=ORIENTED_EDGE('',*,*,#1468,.F.);
#1950=ORIENTED_EDGE('',*,*,#1469,.F.);
#1951=ORIENTED_EDGE('',*,*,#1470,.F.);
#1952=ORIENTED_EDGE('',*,*,#1471,.T.);
#1953=ORIENTED_EDGE('',*,*,#1472,.F.);
#1954=ORIENTED_EDGE('',*,*,#1467,.F.);
#1955=ORIENTED_EDGE('',*,*,#1473,.F.);
#1956=ORIENTED_EDGE('',*,*,#1474,.T.);
#1957=ORIENTED_EDGE('',*,*,#1475,.F.);
#1958=ORIENTED_EDGE('',*,*,#1471,.F.);
#1959=ORIENTED_EDGE('',*,*,#1476,.F.);
#1960=ORIENTED_EDGE('',*,*,#1477,.T.);
#1961=ORIENTED_EDGE('',*,*,#1478,.F.);
#1962=ORIENTED_EDGE('',*,*,#1474,.F.);
#1963=ORIENTED_EDGE('',*,*,#1479,.F.);
#1964=ORIENTED_EDGE('',*,*,#1480,.T.);
#1965=ORIENTED_EDGE('',*,*,#1481,.F.);
#1966=ORIENTED_EDGE('',*,*,#1477,.F.);
#1967=ORIENTED_EDGE('',*,*,#1482,.F.);
#1968=ORIENTED_EDGE('',*,*,#1483,.T.);
#1969=ORIENTED_EDGE('',*,*,#1484,.F.);
#1970=ORIENTED_EDGE('',*,*,#1480,.F.);
#1971=ORIENTED_EDGE('',*,*,#1485,.F.);
#1972=ORIENTED_EDGE('',*,*,#1486,.T.);
#1973=ORIENTED_EDGE('',*,*,#1487,.F.);
#1974=ORIENTED_EDGE('',*,*,#1483,.F.);
#1975=ORIENTED_EDGE('',*,*,#1488,.F.);
#1976=ORIENTED_EDGE('',*,*,#1489,.T.);
#1977=ORIENTED_EDGE('',*,*,#1490,.F.);
#1978=ORIENTED_EDGE('',*,*,#1486,.F.);
#1979=ORIENTED_EDGE('',*,*,#1491,.F.);
#1980=ORIENTED_EDGE('',*,*,#1492,.F.);
#1981=ORIENTED_EDGE('',*,*,#1493,.F.);
#1982=ORIENTED_EDGE('',*,*,#1489,.F.);
#1983=ORIENTED_EDGE('',*,*,#1494,.F.);
#1984=ORIENTED_EDGE('',*,*,#1495,.T.);
#1985=ORIENTED_EDGE('',*,*,#1496,.F.);
#1986=ORIENTED_EDGE('',*,*,#1495,.F.);
#1987=ORIENTED_EDGE('',*,*,#1408,.T.);
#1988=ORIENTED_EDGE('',*,*,#1497,.T.);
#1989=ORIENTED_EDGE('',*,*,#1498,.T.);
#1990=ORIENTED_EDGE('',*,*,#1499,.F.);
#1991=ORIENTED_EDGE('',*,*,#1385,.T.);
#1992=ORIENTED_EDGE('',*,*,#1500,.F.);
#1993=ORIENTED_EDGE('',*,*,#1501,.F.);
#1994=ORIENTED_EDGE('',*,*,#1502,.T.);
#1995=ORIENTED_EDGE('',*,*,#1436,.T.);
#1996=ORIENTED_EDGE('',*,*,#1503,.T.);
#1997=ORIENTED_EDGE('',*,*,#1501,.T.);
#1998=ORIENTED_EDGE('',*,*,#1504,.F.);
#1999=ORIENTED_EDGE('',*,*,#1413,.T.);
#2000=ORIENTED_EDGE('',*,*,#1505,.F.);
#2001=ORIENTED_EDGE('',*,*,#1506,.F.);
#2002=ORIENTED_EDGE('',*,*,#1507,.T.);
#2003=ORIENTED_EDGE('',*,*,#1464,.T.);
#2004=ORIENTED_EDGE('',*,*,#1508,.T.);
#2005=ORIENTED_EDGE('',*,*,#1506,.T.);
#2006=ORIENTED_EDGE('',*,*,#1509,.F.);
#2007=ORIENTED_EDGE('',*,*,#1441,.T.);
#2008=ORIENTED_EDGE('',*,*,#1510,.F.);
#2009=ORIENTED_EDGE('',*,*,#1511,.F.);
#2010=ORIENTED_EDGE('',*,*,#1512,.T.);
#2011=ORIENTED_EDGE('',*,*,#1492,.T.);
#2012=ORIENTED_EDGE('',*,*,#1513,.T.);
#2013=ORIENTED_EDGE('',*,*,#1511,.T.);
#2014=ORIENTED_EDGE('',*,*,#1514,.F.);
#2015=ORIENTED_EDGE('',*,*,#1469,.T.);
#2016=ORIENTED_EDGE('',*,*,#1515,.F.);
#2017=ORIENTED_EDGE('',*,*,#1498,.F.);
#2018=ORIENTED_EDGE('',*,*,#1516,.T.);
#2019=ORIENTED_EDGE('',*,*,#1384,.T.);
#2020=ORIENTED_EDGE('',*,*,#1388,.T.);
#2021=ORIENTED_EDGE('',*,*,#1391,.T.);
#2022=ORIENTED_EDGE('',*,*,#1394,.T.);
#2023=ORIENTED_EDGE('',*,*,#1397,.T.);
#2024=ORIENTED_EDGE('',*,*,#1400,.T.);
#2025=ORIENTED_EDGE('',*,*,#1403,.T.);
#2026=ORIENTED_EDGE('',*,*,#1406,.T.);
#2027=ORIENTED_EDGE('',*,*,#1409,.T.);
#2028=ORIENTED_EDGE('',*,*,#1499,.T.);
#2029=ORIENTED_EDGE('',*,*,#1515,.T.);
#2030=ORIENTED_EDGE('',*,*,#1468,.T.);
#2031=ORIENTED_EDGE('',*,*,#1472,.T.);
#2032=ORIENTED_EDGE('',*,*,#1475,.T.);
#2033=ORIENTED_EDGE('',*,*,#1478,.T.);
#2034=ORIENTED_EDGE('',*,*,#1481,.T.);
#2035=ORIENTED_EDGE('',*,*,#1484,.T.);
#2036=ORIENTED_EDGE('',*,*,#1487,.T.);
#2037=ORIENTED_EDGE('',*,*,#1490,.T.);
#2038=ORIENTED_EDGE('',*,*,#1493,.T.);
#2039=ORIENTED_EDGE('',*,*,#1514,.T.);
#2040=ORIENTED_EDGE('',*,*,#1510,.T.);
#2041=ORIENTED_EDGE('',*,*,#1440,.T.);
#2042=ORIENTED_EDGE('',*,*,#1444,.T.);
#2043=ORIENTED_EDGE('',*,*,#1447,.T.);
#2044=ORIENTED_EDGE('',*,*,#1450,.T.);
#2045=ORIENTED_EDGE('',*,*,#1453,.T.);
#2046=ORIENTED_EDGE('',*,*,#1456,.T.);
#2047=ORIENTED_EDGE('',*,*,#1459,.T.);
#2048=ORIENTED_EDGE('',*,*,#1462,.T.);
#2049=ORIENTED_EDGE('',*,*,#1465,.T.);
#2050=ORIENTED_EDGE('',*,*,#1509,.T.);
#2051=ORIENTED_EDGE('',*,*,#1505,.T.);
#2052=ORIENTED_EDGE('',*,*,#1412,.T.);
#2053=ORIENTED_EDGE('',*,*,#1416,.T.);
#2054=ORIENTED_EDGE('',*,*,#1419,.T.);
#2055=ORIENTED_EDGE('',*,*,#1422,.T.);
#2056=ORIENTED_EDGE('',*,*,#1425,.T.);
#2057=ORIENTED_EDGE('',*,*,#1428,.T.);
#2058=ORIENTED_EDGE('',*,*,#1431,.T.);
#2059=ORIENTED_EDGE('',*,*,#1434,.T.);
#2060=ORIENTED_EDGE('',*,*,#1437,.T.);
#2061=ORIENTED_EDGE('',*,*,#1504,.T.);
#2062=ORIENTED_EDGE('',*,*,#1500,.T.);
#2063=ORIENTED_EDGE('',*,*,#1496,.T.);
#2064=ORIENTED_EDGE('',*,*,#1382,.T.);
#2065=ORIENTED_EDGE('',*,*,#1502,.F.);
#2066=ORIENTED_EDGE('',*,*,#1503,.F.);
#2067=ORIENTED_EDGE('',*,*,#1435,.T.);
#2068=ORIENTED_EDGE('',*,*,#1432,.T.);
#2069=ORIENTED_EDGE('',*,*,#1429,.T.);
#2070=ORIENTED_EDGE('',*,*,#1426,.T.);
#2071=ORIENTED_EDGE('',*,*,#1423,.T.);
#2072=ORIENTED_EDGE('',*,*,#1420,.T.);
#2073=ORIENTED_EDGE('',*,*,#1417,.T.);
#2074=ORIENTED_EDGE('',*,*,#1414,.T.);
#2075=ORIENTED_EDGE('',*,*,#1410,.T.);
#2076=ORIENTED_EDGE('',*,*,#1507,.F.);
#2077=ORIENTED_EDGE('',*,*,#1508,.F.);
#2078=ORIENTED_EDGE('',*,*,#1463,.T.);
#2079=ORIENTED_EDGE('',*,*,#1460,.T.);
#2080=ORIENTED_EDGE('',*,*,#1457,.T.);
#2081=ORIENTED_EDGE('',*,*,#1454,.T.);
#2082=ORIENTED_EDGE('',*,*,#1451,.T.);
#2083=ORIENTED_EDGE('',*,*,#1448,.T.);
#2084=ORIENTED_EDGE('',*,*,#1445,.T.);
#2085=ORIENTED_EDGE('',*,*,#1442,.T.);
#2086=ORIENTED_EDGE('',*,*,#1438,.T.);
#2087=ORIENTED_EDGE('',*,*,#1512,.F.);
#2088=ORIENTED_EDGE('',*,*,#1513,.F.);
#2089=ORIENTED_EDGE('',*,*,#1491,.T.);
#2090=ORIENTED_EDGE('',*,*,#1488,.T.);
#2091=ORIENTED_EDGE('',*,*,#1485,.T.);
#2092=ORIENTED_EDGE('',*,*,#1482,.T.);
#2093=ORIENTED_EDGE('',*,*,#1479,.T.);
#2094=ORIENTED_EDGE('',*,*,#1476,.T.);
#2095=ORIENTED_EDGE('',*,*,#1473,.T.);
#2096=ORIENTED_EDGE('',*,*,#1470,.T.);
#2097=ORIENTED_EDGE('',*,*,#1466,.T.);
#2098=ORIENTED_EDGE('',*,*,#1516,.F.);
#2099=ORIENTED_EDGE('',*,*,#1497,.F.);
#2100=ORIENTED_EDGE('',*,*,#1407,.T.);
#2101=ORIENTED_EDGE('',*,*,#1404,.T.);
#2102=ORIENTED_EDGE('',*,*,#1401,.T.);
#2103=ORIENTED_EDGE('',*,*,#1398,.T.);
#2104=ORIENTED_EDGE('',*,*,#1395,.T.);
#2105=ORIENTED_EDGE('',*,*,#1392,.T.);
#2106=ORIENTED_EDGE('',*,*,#1389,.T.);
#2107=ORIENTED_EDGE('',*,*,#1386,.T.);
#2108=ORIENTED_EDGE('',*,*,#1494,.T.);
#2117=CYLINDRICAL_SURFACE('',#2486,0.21);
#2190=ADVANCED_FACE('',(#290),#172,.F.);
#2191=ADVANCED_FACE('',(#291),#173,.F.);
#2192=ADVANCED_FACE('',(#292),#174,.F.);
#2193=ADVANCED_FACE('',(#293),#175,.F.);
#2194=ADVANCED_FACE('',(#294),#176,.F.);
#2195=ADVANCED_FACE('',(#295),#177,.F.);
#2196=ADVANCED_FACE('',(#296),#178,.F.);
#2197=ADVANCED_FACE('',(#297),#179,.F.);
#2198=ADVANCED_FACE('',(#298),#180,.F.);
#2199=ADVANCED_FACE('',(#299),#181,.F.);
#2200=ADVANCED_FACE('',(#300),#182,.F.);
#2201=ADVANCED_FACE('',(#301),#183,.F.);
#2202=ADVANCED_FACE('',(#302),#184,.F.);
#2203=ADVANCED_FACE('',(#303),#185,.F.);
#2204=ADVANCED_FACE('',(#304),#186,.F.);
#2205=ADVANCED_FACE('',(#305),#187,.F.);
#2206=ADVANCED_FACE('',(#306),#188,.F.);
#2207=ADVANCED_FACE('',(#307),#189,.F.);
#2208=ADVANCED_FACE('',(#308),#190,.F.);
#2209=ADVANCED_FACE('',(#309),#191,.F.);
#2210=ADVANCED_FACE('',(#310),#192,.F.);
#2211=ADVANCED_FACE('',(#311),#193,.F.);
#2212=ADVANCED_FACE('',(#312),#194,.F.);
#2213=ADVANCED_FACE('',(#313),#195,.F.);
#2214=ADVANCED_FACE('',(#314),#196,.F.);
#2215=ADVANCED_FACE('',(#315),#197,.F.);
#2216=ADVANCED_FACE('',(#316),#198,.F.);
#2217=ADVANCED_FACE('',(#317),#199,.F.);
#2218=ADVANCED_FACE('',(#318),#200,.F.);
#2219=ADVANCED_FACE('',(#319),#201,.F.);
#2220=ADVANCED_FACE('',(#320),#202,.F.);
#2221=ADVANCED_FACE('',(#321),#203,.F.);
#2222=ADVANCED_FACE('',(#322),#204,.F.);
#2223=ADVANCED_FACE('',(#323),#205,.F.);
#2224=ADVANCED_FACE('',(#324),#206,.F.);
#2225=ADVANCED_FACE('',(#325),#207,.F.);
#2226=ADVANCED_FACE('',(#326),#2117,.F.);
#2227=ADVANCED_FACE('',(#327),#208,.T.);
#2228=ADVANCED_FACE('',(#328),#209,.T.);
#2229=ADVANCED_FACE('',(#329),#210,.T.);
#2230=ADVANCED_FACE('',(#330),#211,.T.);
#2231=ADVANCED_FACE('',(#331),#212,.T.);
#2232=ADVANCED_FACE('',(#332),#213,.T.);
#2233=ADVANCED_FACE('',(#333),#214,.T.);
#2234=ADVANCED_FACE('',(#334),#215,.T.);
#2235=ADVANCED_FACE('',(#335,#113),#216,.T.);
#2236=ADVANCED_FACE('',(#336,#114),#217,.F.);
#2244=CLOSED_SHELL('',(#2190,#2191,#2192,#2193,#2194,#2195,#2196,#2197,
#2198,#2199,#2200,#2201,#2202,#2203,#2204,#2205,#2206,#2207,#2208,#2209,
#2210,#2211,#2212,#2213,#2214,#2215,#2216,#2217,#2218,#2219,#2220,#2221,
#2222,#2223,#2224,#2225,#2226,#2227,#2228,#2229,#2230,#2231,#2232,#2233,
#2234,#2235,#2236));
#2449=AXIS2_PLACEMENT_3D('',#3472,#2863,#2864);
#2450=AXIS2_PLACEMENT_3D('',#3473,#2865,#2866);
#2451=AXIS2_PLACEMENT_3D('',#3482,#2871,#2872);
#2452=AXIS2_PLACEMENT_3D('',#3488,#2876,#2877);
#2453=AXIS2_PLACEMENT_3D('',#3494,#2881,#2882);
#2454=AXIS2_PLACEMENT_3D('',#3500,#2886,#2887);
#2455=AXIS2_PLACEMENT_3D('',#3506,#2891,#2892);
#2456=AXIS2_PLACEMENT_3D('',#3512,#2896,#2897);
#2457=AXIS2_PLACEMENT_3D('',#3518,#2901,#2902);
#2458=AXIS2_PLACEMENT_3D('',#3524,#2906,#2907);
#2459=AXIS2_PLACEMENT_3D('',#3530,#2911,#2912);
#2460=AXIS2_PLACEMENT_3D('',#3539,#2917,#2918);
#2461=AXIS2_PLACEMENT_3D('',#3545,#2922,#2923);
#2462=AXIS2_PLACEMENT_3D('',#3551,#2927,#2928);
#2463=AXIS2_PLACEMENT_3D('',#3557,#2932,#2933);
#2464=AXIS2_PLACEMENT_3D('',#3563,#2937,#2938);
#2465=AXIS2_PLACEMENT_3D('',#3569,#2942,#2943);
#2466=AXIS2_PLACEMENT_3D('',#3575,#2947,#2948);
#2467=AXIS2_PLACEMENT_3D('',#3581,#2952,#2953);
#2468=AXIS2_PLACEMENT_3D('',#3587,#2957,#2958);
#2469=AXIS2_PLACEMENT_3D('',#3596,#2963,#2964);
#2470=AXIS2_PLACEMENT_3D('',#3602,#2968,#2969);
#2471=AXIS2_PLACEMENT_3D('',#3608,#2973,#2974);
#2472=AXIS2_PLACEMENT_3D('',#3614,#2978,#2979);
#2473=AXIS2_PLACEMENT_3D('',#3620,#2983,#2984);
#2474=AXIS2_PLACEMENT_3D('',#3626,#2988,#2989);
#2475=AXIS2_PLACEMENT_3D('',#3632,#2993,#2994);
#2476=AXIS2_PLACEMENT_3D('',#3638,#2998,#2999);
#2477=AXIS2_PLACEMENT_3D('',#3644,#3003,#3004);
#2478=AXIS2_PLACEMENT_3D('',#3653,#3009,#3010);
#2479=AXIS2_PLACEMENT_3D('',#3659,#3014,#3015);
#2480=AXIS2_PLACEMENT_3D('',#3665,#3019,#3020);
#2481=AXIS2_PLACEMENT_3D('',#3671,#3024,#3025);
#2482=AXIS2_PLACEMENT_3D('',#3677,#3029,#3030);
#2483=AXIS2_PLACEMENT_3D('',#3683,#3034,#3035);
#2484=AXIS2_PLACEMENT_3D('',#3689,#3039,#3040);
#2485=AXIS2_PLACEMENT_3D('',#3695,#3044,#3045);
#2486=AXIS2_PLACEMENT_3D('',#3701,#3049,#3050);
#2487=AXIS2_PLACEMENT_3D('',#3703,#3051,#3052);
#2488=AXIS2_PLACEMENT_3D('',#3706,#3054,#3055);
#2489=AXIS2_PLACEMENT_3D('',#3707,#3056,#3057);
#2490=AXIS2_PLACEMENT_3D('',#3713,#3061,#3062);
#2491=AXIS2_PLACEMENT_3D('',#3719,#3066,#3067);
#2492=AXIS2_PLACEMENT_3D('',#3722,#3070,#3071);
#2493=AXIS2_PLACEMENT_3D('',#3728,#3075,#3076);
#2494=AXIS2_PLACEMENT_3D('',#3731,#3079,#3080);
#2495=AXIS2_PLACEMENT_3D('',#3737,#3084,#3085);
#2496=AXIS2_PLACEMENT_3D('',#3740,#3088,#3089);
#2497=AXIS2_PLACEMENT_3D('',#3743,#3092,#3093);
#2498=AXIS2_PLACEMENT_3D('',#3744,#3094,#3095);
#2863=DIRECTION('axis',(0.,0.,1.));
#2864=DIRECTION('refdir',(1.,0.,0.));
#2865=DIRECTION('center_axis',(0.,0.,-1.));
#2866=DIRECTION('ref_axis',(0.,1.,0.));
#2867=DIRECTION('',(0.,1.,0.));
#2868=DIRECTION('',(1.,0.,0.));
#2869=DIRECTION('',(0.,-1.,0.));
#2870=DIRECTION('',(1.,0.,0.));
#2871=DIRECTION('center_axis',(0.,1.,-8.88178419700125E-16));
#2872=DIRECTION('ref_axis',(0.,8.88178419700125E-16,1.));
#2873=DIRECTION('',(0.,8.88178419700125E-16,1.));
#2874=DIRECTION('',(1.,0.,0.));
#2875=DIRECTION('',(0.,-8.88178419700125E-16,-1.));
#2876=DIRECTION('center_axis',(0.,-7.40148683083439E-16,-1.));
#2877=DIRECTION('ref_axis',(0.,1.,-7.40148683083439E-16));
#2878=DIRECTION('',(0.,1.,-7.40148683083439E-16));
#2879=DIRECTION('',(1.,0.,0.));
#2880=DIRECTION('',(0.,-1.,7.40148683083439E-16));
#2881=DIRECTION('center_axis',(0.,-0.707106781186547,-0.707106781186548));
#2882=DIRECTION('ref_axis',(0.,0.707106781186548,-0.707106781186547));
#2883=DIRECTION('',(0.,0.707106781186548,-0.707106781186547));
#2884=DIRECTION('',(1.,0.,0.));
#2885=DIRECTION('',(0.,-0.707106781186548,0.707106781186547));
#2886=DIRECTION('center_axis',(0.,-1.,2.77555756156289E-16));
#2887=DIRECTION('ref_axis',(0.,-2.77555756156289E-16,-1.));
#2888=DIRECTION('',(0.,-2.77555756156289E-16,-1.));
#2889=DIRECTION('',(1.,0.,0.));
#2890=DIRECTION('',(0.,2.77555756156289E-16,1.));
#2891=DIRECTION('center_axis',(0.,-0.707106781186547,0.707106781186548));
#2892=DIRECTION('ref_axis',(0.,-0.707106781186548,-0.707106781186547));
#2893=DIRECTION('',(0.,-0.707106781186548,-0.707106781186547));
#2894=DIRECTION('',(1.,0.,0.));
#2895=DIRECTION('',(0.,0.707106781186548,0.707106781186547));
#2896=DIRECTION('center_axis',(0.,7.40148683083438E-16,1.));
#2897=DIRECTION('ref_axis',(0.,-1.,7.40148683083438E-16));
#2898=DIRECTION('',(0.,-1.,7.40148683083438E-16));
#2899=DIRECTION('',(1.,0.,0.));
#2900=DIRECTION('',(0.,1.,-7.40148683083438E-16));
#2901=DIRECTION('center_axis',(0.,1.,-4.44089209850063E-16));
#2902=DIRECTION('ref_axis',(0.,4.44089209850063E-16,1.));
#2903=DIRECTION('',(0.,4.44089209850063E-16,1.));
#2904=DIRECTION('',(1.,0.,0.));
#2905=DIRECTION('',(0.,-4.44089209850063E-16,-1.));
#2906=DIRECTION('center_axis',(0.,2.41352831440251E-16,1.));
#2907=DIRECTION('ref_axis',(0.,-1.,2.41352831440251E-16));
#2908=DIRECTION('',(0.,-1.,2.41352831440251E-16));
#2909=DIRECTION('',(-1.,0.,0.));
#2910=DIRECTION('',(0.,1.,-2.41352831440251E-16));
#2911=DIRECTION('center_axis',(0.,-1.,2.41352831440251E-16));
#2912=DIRECTION('ref_axis',(0.,-2.41352831440251E-16,-1.));
#2913=DIRECTION('',(0.,-2.41352831440251E-16,-1.));
#2914=DIRECTION('',(1.,0.,0.));
#2915=DIRECTION('',(0.,2.41352831440251E-16,1.));
#2916=DIRECTION('',(1.,0.,0.));
#2917=DIRECTION('center_axis',(0.,0.,-1.));
#2918=DIRECTION('ref_axis',(0.,1.,0.));
#2919=DIRECTION('',(0.,1.,0.));
#2920=DIRECTION('',(1.,0.,0.));
#2921=DIRECTION('',(0.,-1.,0.));
#2922=DIRECTION('center_axis',(0.,-1.,0.));
#2923=DIRECTION('ref_axis',(0.,0.,-1.));
#2924=DIRECTION('',(0.,0.,-1.));
#2925=DIRECTION('',(1.,0.,0.));
#2926=DIRECTION('',(0.,0.,1.));
#2927=DIRECTION('center_axis',(0.,-0.707106781186547,0.707106781186548));
#2928=DIRECTION('ref_axis',(0.,-0.707106781186548,-0.707106781186547));
#2929=DIRECTION('',(0.,-0.707106781186548,-0.707106781186547));
#2930=DIRECTION('',(1.,0.,0.));
#2931=DIRECTION('',(0.,0.707106781186548,0.707106781186547));
#2932=DIRECTION('center_axis',(0.,0.,1.));
#2933=DIRECTION('ref_axis',(0.,-1.,0.));
#2934=DIRECTION('',(0.,-1.,0.));
#2935=DIRECTION('',(1.,0.,0.));
#2936=DIRECTION('',(0.,1.,0.));
#2937=DIRECTION('center_axis',(0.,0.707106781186548,0.707106781186547));
#2938=DIRECTION('ref_axis',(0.,-0.707106781186547,0.707106781186548));
#2939=DIRECTION('',(0.,-0.707106781186547,0.707106781186548));
#2940=DIRECTION('',(1.,0.,0.));
#2941=DIRECTION('',(0.,0.707106781186547,-0.707106781186548));
#2942=DIRECTION('center_axis',(0.,1.,0.));
#2943=DIRECTION('ref_axis',(0.,0.,1.));
#2944=DIRECTION('',(0.,0.,1.));
#2945=DIRECTION('',(1.,0.,0.));
#2946=DIRECTION('',(0.,0.,-1.));
#2947=DIRECTION('center_axis',(0.,0.,-1.));
#2948=DIRECTION('ref_axis',(0.,1.,0.));
#2949=DIRECTION('',(0.,1.,0.));
#2950=DIRECTION('',(1.,0.,0.));
#2951=DIRECTION('',(0.,-1.,0.));
#2952=DIRECTION('center_axis',(0.,1.,-2.41352831440251E-16));
#2953=DIRECTION('ref_axis',(0.,2.41352831440251E-16,1.));
#2954=DIRECTION('',(0.,2.41352831440251E-16,1.));
#2955=DIRECTION('',(-1.,0.,0.));
#2956=DIRECTION('',(0.,-2.41352831440251E-16,-1.));
#2957=DIRECTION('center_axis',(0.,0.,1.));
#2958=DIRECTION('ref_axis',(0.,-1.,0.));
#2959=DIRECTION('',(0.,-1.,0.));
#2960=DIRECTION('',(1.,0.,0.));
#2961=DIRECTION('',(0.,1.,0.));
#2962=DIRECTION('',(1.,0.,0.));
#2963=DIRECTION('center_axis',(0.,-1.,0.));
#2964=DIRECTION('ref_axis',(0.,0.,-1.));
#2965=DIRECTION('',(0.,0.,-1.));
#2966=DIRECTION('',(1.,0.,0.));
#2967=DIRECTION('',(0.,0.,1.));
#2968=DIRECTION('center_axis',(0.,0.,1.));
#2969=DIRECTION('ref_axis',(0.,-1.,0.));
#2970=DIRECTION('',(0.,-1.,0.));
#2971=DIRECTION('',(1.,0.,0.));
#2972=DIRECTION('',(0.,1.,0.));
#2973=DIRECTION('center_axis',(0.,0.707106781186548,0.707106781186548));
#2974=DIRECTION('ref_axis',(0.,-0.707106781186548,0.707106781186548));
#2975=DIRECTION('',(0.,-0.707106781186548,0.707106781186548));
#2976=DIRECTION('',(1.,0.,0.));
#2977=DIRECTION('',(0.,0.707106781186548,-0.707106781186548));
#2978=DIRECTION('center_axis',(0.,1.,0.));
#2979=DIRECTION('ref_axis',(0.,0.,1.));
#2980=DIRECTION('',(0.,0.,1.));
#2981=DIRECTION('',(1.,0.,0.));
#2982=DIRECTION('',(0.,0.,-1.));
#2983=DIRECTION('center_axis',(0.,0.707106781186548,-0.707106781186547));
#2984=DIRECTION('ref_axis',(0.,0.707106781186547,0.707106781186548));
#2985=DIRECTION('',(0.,0.707106781186547,0.707106781186548));
#2986=DIRECTION('',(1.,0.,0.));
#2987=DIRECTION('',(0.,-0.707106781186547,-0.707106781186548));
#2988=DIRECTION('center_axis',(0.,-7.40148683083438E-16,-1.));
#2989=DIRECTION('ref_axis',(0.,1.,-7.40148683083438E-16));
#2990=DIRECTION('',(0.,1.,-7.40148683083438E-16));
#2991=DIRECTION('',(1.,0.,0.));
#2992=DIRECTION('',(0.,-1.,7.40148683083438E-16));
#2993=DIRECTION('center_axis',(0.,-1.,0.));
#2994=DIRECTION('ref_axis',(0.,0.,-1.));
#2995=DIRECTION('',(0.,0.,-1.));
#2996=DIRECTION('',(1.,0.,0.));
#2997=DIRECTION('',(0.,0.,1.));
#2998=DIRECTION('center_axis',(0.,0.,-1.));
#2999=DIRECTION('ref_axis',(0.,1.,0.));
#3000=DIRECTION('',(0.,1.,0.));
#3001=DIRECTION('',(-1.,0.,0.));
#3002=DIRECTION('',(0.,-1.,0.));
#3003=DIRECTION('center_axis',(0.,1.,0.));
#3004=DIRECTION('ref_axis',(0.,0.,1.));
#3005=DIRECTION('',(0.,0.,1.));
#3006=DIRECTION('',(1.,0.,0.));
#3007=DIRECTION('',(0.,0.,-1.));
#3008=DIRECTION('',(1.,0.,0.));
#3009=DIRECTION('center_axis',(0.,0.,1.));
#3010=DIRECTION('ref_axis',(0.,-1.,0.));
#3011=DIRECTION('',(0.,-1.,0.));
#3012=DIRECTION('',(1.,0.,0.));
#3013=DIRECTION('',(0.,1.,0.));
#3014=DIRECTION('center_axis',(0.,1.,0.));
#3015=DIRECTION('ref_axis',(0.,0.,1.));
#3016=DIRECTION('',(0.,0.,1.));
#3017=DIRECTION('',(1.,0.,0.));
#3018=DIRECTION('',(0.,0.,-1.));
#3019=DIRECTION('center_axis',(0.,0.707106781186547,-0.707106781186548));
#3020=DIRECTION('ref_axis',(0.,0.707106781186548,0.707106781186547));
#3021=DIRECTION('',(0.,0.707106781186548,0.707106781186547));
#3022=DIRECTION('',(1.,0.,0.));
#3023=DIRECTION('',(0.,-0.707106781186548,-0.707106781186547));
#3024=DIRECTION('center_axis',(0.,0.,-1.));
#3025=DIRECTION('ref_axis',(0.,1.,0.));
#3026=DIRECTION('',(0.,1.,0.));
#3027=DIRECTION('',(1.,0.,0.));
#3028=DIRECTION('',(0.,-1.,0.));
#3029=DIRECTION('center_axis',(0.,-0.707106781186547,-0.707106781186548));
#3030=DIRECTION('ref_axis',(0.,0.707106781186548,-0.707106781186547));
#3031=DIRECTION('',(0.,0.707106781186548,-0.707106781186547));
#3032=DIRECTION('',(1.,0.,0.));
#3033=DIRECTION('',(0.,-0.707106781186548,0.707106781186547));
#3034=DIRECTION('center_axis',(0.,-1.,0.));
#3035=DIRECTION('ref_axis',(0.,0.,-1.));
#3036=DIRECTION('',(0.,0.,-1.));
#3037=DIRECTION('',(1.,0.,0.));
#3038=DIRECTION('',(0.,0.,1.));
#3039=DIRECTION('center_axis',(0.,0.,1.));
#3040=DIRECTION('ref_axis',(0.,-1.,0.));
#3041=DIRECTION('',(0.,-1.,0.));
#3042=DIRECTION('',(1.,0.,0.));
#3043=DIRECTION('',(0.,1.,0.));
#3044=DIRECTION('center_axis',(0.,-1.,0.));
#3045=DIRECTION('ref_axis',(0.,0.,-1.));
#3046=DIRECTION('',(0.,0.,-1.));
#3047=DIRECTION('',(-1.,0.,0.));
#3048=DIRECTION('',(0.,0.,1.));
#3049=DIRECTION('center_axis',(1.,0.,0.));
#3050=DIRECTION('ref_axis',(0.,0.,-1.));
#3051=DIRECTION('center_axis',(1.,0.,0.));
#3052=DIRECTION('ref_axis',(0.,0.,-1.));
#3053=DIRECTION('',(1.,0.,0.));
#3054=DIRECTION('center_axis',(-1.,0.,0.));
#3055=DIRECTION('ref_axis',(0.,0.,-1.));
#3056=DIRECTION('center_axis',(0.,1.,0.));
#3057=DIRECTION('ref_axis',(0.,0.,1.));
#3058=DIRECTION('',(0.,0.,1.));
#3059=DIRECTION('',(1.,0.,0.));
#3060=DIRECTION('',(0.,0.,1.));
#3061=DIRECTION('center_axis',(0.,1.,0.));
#3062=DIRECTION('ref_axis',(0.,0.,1.));
#3063=DIRECTION('',(0.,0.,1.));
#3064=DIRECTION('',(1.,0.,0.));
#3065=DIRECTION('',(0.,0.,1.));
#3066=DIRECTION('center_axis',(0.,0.,-1.));
#3067=DIRECTION('ref_axis',(0.,1.,0.));
#3068=DIRECTION('',(0.,1.,0.));
#3069=DIRECTION('',(0.,1.,0.));
#3070=DIRECTION('center_axis',(0.,0.,-1.));
#3071=DIRECTION('ref_axis',(0.,1.,0.));
#3072=DIRECTION('',(0.,1.,0.));
#3073=DIRECTION('',(1.,0.,0.));
#3074=DIRECTION('',(0.,1.,0.));
#3075=DIRECTION('center_axis',(0.,-1.,0.));
#3076=DIRECTION('ref_axis',(0.,0.,-1.));
#3077=DIRECTION('',(0.,0.,-1.));
#3078=DIRECTION('',(0.,0.,-1.));
#3079=DIRECTION('center_axis',(0.,-1.,0.));
#3080=DIRECTION('ref_axis',(0.,0.,-1.));
#3081=DIRECTION('',(0.,0.,-1.));
#3082=DIRECTION('',(1.,0.,0.));
#3083=DIRECTION('',(0.,0.,-1.));
#3084=DIRECTION('center_axis',(0.,0.,1.));
#3085=DIRECTION('ref_axis',(0.,-1.,0.));
#3086=DIRECTION('',(0.,-1.,0.));
#3087=DIRECTION('',(0.,-1.,0.));
#3088=DIRECTION('center_axis',(0.,0.,1.));
#3089=DIRECTION('ref_axis',(0.,-1.,0.));
#3090=DIRECTION('',(0.,-1.,0.));
#3091=DIRECTION('',(0.,-1.,0.));
#3092=DIRECTION('center_axis',(1.,0.,0.));
#3093=DIRECTION('ref_axis',(0.,0.,-1.));
#3094=DIRECTION('center_axis',(1.,0.,0.));
#3095=DIRECTION('ref_axis',(0.,0.,-1.));
#3472=CARTESIAN_POINT('',(0.,0.,0.));
#3473=CARTESIAN_POINT('Origin',(-0.1,0.82,-0.3));
#3474=CARTESIAN_POINT('',(0.,0.82,-0.3));
#3475=CARTESIAN_POINT('',(0.,1.,-0.3));
#3476=CARTESIAN_POINT('',(0.,0.41,-0.3));
#3477=CARTESIAN_POINT('',(30.,0.82,-0.3));
#3478=CARTESIAN_POINT('',(-0.1,0.82,-0.3));
#3479=CARTESIAN_POINT('',(30.,1.,-0.3));
#3480=CARTESIAN_POINT('',(30.,0.41,-0.3));
#3481=CARTESIAN_POINT('',(-0.05,1.,-0.3));
#3482=CARTESIAN_POINT('Origin',(-0.1,0.82,-0.55));
#3483=CARTESIAN_POINT('',(0.,0.82,-0.55));
#3484=CARTESIAN_POINT('',(0.,0.82,-0.275));
#3485=CARTESIAN_POINT('',(30.,0.82,-0.55));
#3486=CARTESIAN_POINT('',(-0.1,0.82,-0.55));
#3487=CARTESIAN_POINT('',(30.,0.82,-0.275));
#3488=CARTESIAN_POINT('Origin',(-0.1,0.67,-0.55));
#3489=CARTESIAN_POINT('',(0.,0.67,-0.55));
#3490=CARTESIAN_POINT('',(0.,0.335,-0.55));
#3491=CARTESIAN_POINT('',(30.,0.67,-0.55));
#3492=CARTESIAN_POINT('',(-0.1,0.67,-0.55));
#3493=CARTESIAN_POINT('',(30.,0.335,-0.55));
#3494=CARTESIAN_POINT('Origin',(-0.1,0.42,-0.3));
#3495=CARTESIAN_POINT('',(0.,0.42,-0.3));
#3496=CARTESIAN_POINT('',(0.,0.24,-0.12));
#3497=CARTESIAN_POINT('',(30.,0.42,-0.3));
#3498=CARTESIAN_POINT('',(-0.1,0.42,-0.3));
#3499=CARTESIAN_POINT('',(30.,0.24,-0.12));
#3500=CARTESIAN_POINT('Origin',(-0.1,0.42,0.3));
#3501=CARTESIAN_POINT('',(0.,0.42,0.3));
#3502=CARTESIAN_POINT('',(0.,0.42,0.15));
#3503=CARTESIAN_POINT('',(30.,0.42,0.3));
#3504=CARTESIAN_POINT('',(-0.1,0.42,0.3));
#3505=CARTESIAN_POINT('',(30.,0.42,0.15));
#3506=CARTESIAN_POINT('Origin',(-0.1,0.67,0.55));
#3507=CARTESIAN_POINT('',(0.,0.67,0.55));
#3508=CARTESIAN_POINT('',(6.93889390390723E-18,0.365,0.245));
#3509=CARTESIAN_POINT('',(30.,0.67,0.55));
#3510=CARTESIAN_POINT('',(-0.1,0.67,0.55));
#3511=CARTESIAN_POINT('',(30.,0.365,0.245));
#3512=CARTESIAN_POINT('Origin',(-0.1,0.82,0.55));
#3513=CARTESIAN_POINT('',(0.,0.82,0.55));
#3514=CARTESIAN_POINT('',(0.,0.41,0.55));
#3515=CARTESIAN_POINT('',(30.,0.82,0.55));
#3516=CARTESIAN_POINT('',(-0.1,0.82,0.55));
#3517=CARTESIAN_POINT('',(30.,0.41,0.55));
#3518=CARTESIAN_POINT('Origin',(-0.1,0.82,0.3));
#3519=CARTESIAN_POINT('',(0.,0.82,0.3));
#3520=CARTESIAN_POINT('',(0.,0.82,0.15));
#3521=CARTESIAN_POINT('',(30.,0.82,0.3));
#3522=CARTESIAN_POINT('',(-0.1,0.82,0.3));
#3523=CARTESIAN_POINT('',(30.,0.82,0.15));
#3524=CARTESIAN_POINT('Origin',(-0.1,1.05,0.3));
#3525=CARTESIAN_POINT('',(0.,1.,0.3));
#3526=CARTESIAN_POINT('',(0.,0.525,0.3));
#3527=CARTESIAN_POINT('',(30.,1.,0.3));
#3528=CARTESIAN_POINT('',(-0.05,1.,0.3));
#3529=CARTESIAN_POINT('',(30.,0.525,0.3));
#3530=CARTESIAN_POINT('Origin',(-0.1,-0.3,-0.82));
#3531=CARTESIAN_POINT('',(0.,-0.3,-0.82));
#3532=CARTESIAN_POINT('',(0.,-0.3,-1.));
#3533=CARTESIAN_POINT('',(0.,-0.3,-0.41));
#3534=CARTESIAN_POINT('',(30.,-0.3,-0.82));
#3535=CARTESIAN_POINT('',(-0.1,-0.3,-0.82));
#3536=CARTESIAN_POINT('',(30.,-0.3,-1.));
#3537=CARTESIAN_POINT('',(30.,-0.3,-0.41));
#3538=CARTESIAN_POINT('',(-0.05,-0.3,-1.));
#3539=CARTESIAN_POINT('Origin',(-0.1,-0.55,-0.82));
#3540=CARTESIAN_POINT('',(0.,-0.55,-0.82));
#3541=CARTESIAN_POINT('',(0.,-0.275,-0.82));
#3542=CARTESIAN_POINT('',(30.,-0.55,-0.82));
#3543=CARTESIAN_POINT('',(-0.1,-0.55,-0.82));
#3544=CARTESIAN_POINT('',(30.,-0.275,-0.82));
#3545=CARTESIAN_POINT('Origin',(-0.1,-0.55,-0.67));
#3546=CARTESIAN_POINT('',(0.,-0.55,-0.67));
#3547=CARTESIAN_POINT('',(0.,-0.55,-0.335));
#3548=CARTESIAN_POINT('',(30.,-0.55,-0.67));
#3549=CARTESIAN_POINT('',(-0.1,-0.55,-0.67));
#3550=CARTESIAN_POINT('',(30.,-0.55,-0.335));
#3551=CARTESIAN_POINT('Origin',(-0.1,-0.3,-0.42));
#3552=CARTESIAN_POINT('',(0.,-0.3,-0.42));
#3553=CARTESIAN_POINT('',(0.,-0.12,-0.24));
#3554=CARTESIAN_POINT('',(30.,-0.3,-0.42));
#3555=CARTESIAN_POINT('',(-0.1,-0.3,-0.42));
#3556=CARTESIAN_POINT('',(30.,-0.12,-0.24));
#3557=CARTESIAN_POINT('Origin',(-0.1,0.3,-0.42));
#3558=CARTESIAN_POINT('',(0.,0.3,-0.42));
#3559=CARTESIAN_POINT('',(0.,0.15,-0.42));
#3560=CARTESIAN_POINT('',(30.,0.3,-0.42));
#3561=CARTESIAN_POINT('',(-0.1,0.3,-0.42));
#3562=CARTESIAN_POINT('',(30.,0.15,-0.42));
#3563=CARTESIAN_POINT('Origin',(-0.1,0.55,-0.67));
#3564=CARTESIAN_POINT('',(0.,0.55,-0.67));
#3565=CARTESIAN_POINT('',(0.,0.245,-0.365));
#3566=CARTESIAN_POINT('',(30.,0.55,-0.67));
#3567=CARTESIAN_POINT('',(-0.1,0.55,-0.67));
#3568=CARTESIAN_POINT('',(30.,0.245,-0.365));
#3569=CARTESIAN_POINT('Origin',(-0.1,0.55,-0.82));
#3570=CARTESIAN_POINT('',(0.,0.55,-0.82));
#3571=CARTESIAN_POINT('',(0.,0.55,-0.41));
#3572=CARTESIAN_POINT('',(30.,0.55,-0.82));
#3573=CARTESIAN_POINT('',(-0.1,0.55,-0.82));
#3574=CARTESIAN_POINT('',(30.,0.55,-0.41));
#3575=CARTESIAN_POINT('Origin',(-0.1,0.3,-0.82));
#3576=CARTESIAN_POINT('',(0.,0.3,-0.82));
#3577=CARTESIAN_POINT('',(0.,0.15,-0.82));
#3578=CARTESIAN_POINT('',(30.,0.3,-0.82));
#3579=CARTESIAN_POINT('',(-0.1,0.3,-0.82));
#3580=CARTESIAN_POINT('',(30.,0.15,-0.82));
#3581=CARTESIAN_POINT('Origin',(-0.1,0.3,-1.05));
#3582=CARTESIAN_POINT('',(0.,0.3,-1.));
#3583=CARTESIAN_POINT('',(0.,0.3,-0.525));
#3584=CARTESIAN_POINT('',(30.,0.3,-1.));
#3585=CARTESIAN_POINT('',(-0.05,0.3,-1.));
#3586=CARTESIAN_POINT('',(30.,0.3,-0.525));
#3587=CARTESIAN_POINT('Origin',(-0.1,-0.82,0.3));
#3588=CARTESIAN_POINT('',(0.,-0.82,0.3));
#3589=CARTESIAN_POINT('',(0.,-1.,0.3));
#3590=CARTESIAN_POINT('',(0.,-0.41,0.3));
#3591=CARTESIAN_POINT('',(30.,-0.82,0.3));
#3592=CARTESIAN_POINT('',(-0.1,-0.82,0.3));
#3593=CARTESIAN_POINT('',(30.,-1.,0.3));
#3594=CARTESIAN_POINT('',(30.,-0.41,0.3));
#3595=CARTESIAN_POINT('',(-0.05,-1.,0.3));
#3596=CARTESIAN_POINT('Origin',(-0.1,-0.82,0.55));
#3597=CARTESIAN_POINT('',(0.,-0.82,0.55));
#3598=CARTESIAN_POINT('',(0.,-0.82,0.275));
#3599=CARTESIAN_POINT('',(30.,-0.82,0.55));
#3600=CARTESIAN_POINT('',(-0.1,-0.82,0.55));
#3601=CARTESIAN_POINT('',(30.,-0.82,0.275));
#3602=CARTESIAN_POINT('Origin',(-0.1,-0.67,0.55));
#3603=CARTESIAN_POINT('',(0.,-0.67,0.55));
#3604=CARTESIAN_POINT('',(0.,-0.335,0.55));
#3605=CARTESIAN_POINT('',(30.,-0.67,0.55));
#3606=CARTESIAN_POINT('',(-0.1,-0.67,0.55));
#3607=CARTESIAN_POINT('',(30.,-0.335,0.55));
#3608=CARTESIAN_POINT('Origin',(-0.1,-0.42,0.3));
#3609=CARTESIAN_POINT('',(0.,-0.42,0.3));
#3610=CARTESIAN_POINT('',(-6.93889390390723E-18,-0.24,0.12));
#3611=CARTESIAN_POINT('',(30.,-0.42,0.3));
#3612=CARTESIAN_POINT('',(-0.1,-0.42,0.3));
#3613=CARTESIAN_POINT('',(30.,-0.24,0.12));
#3614=CARTESIAN_POINT('Origin',(-0.1,-0.42,-0.3));
#3615=CARTESIAN_POINT('',(0.,-0.42,-0.3));
#3616=CARTESIAN_POINT('',(0.,-0.42,-0.15));
#3617=CARTESIAN_POINT('',(30.,-0.42,-0.3));
#3618=CARTESIAN_POINT('',(-0.1,-0.42,-0.3));
#3619=CARTESIAN_POINT('',(30.,-0.42,-0.15));
#3620=CARTESIAN_POINT('Origin',(-0.1,-0.67,-0.55));
#3621=CARTESIAN_POINT('',(0.,-0.67,-0.55));
#3622=CARTESIAN_POINT('',(0.,-0.365,-0.245));
#3623=CARTESIAN_POINT('',(30.,-0.67,-0.55));
#3624=CARTESIAN_POINT('',(-0.1,-0.67,-0.55));
#3625=CARTESIAN_POINT('',(30.,-0.365,-0.245));
#3626=CARTESIAN_POINT('Origin',(-0.1,-0.82,-0.55));
#3627=CARTESIAN_POINT('',(0.,-0.82,-0.55));
#3628=CARTESIAN_POINT('',(0.,-0.41,-0.55));
#3629=CARTESIAN_POINT('',(30.,-0.82,-0.55));
#3630=CARTESIAN_POINT('',(-0.1,-0.82,-0.55));
#3631=CARTESIAN_POINT('',(30.,-0.41,-0.55));
#3632=CARTESIAN_POINT('Origin',(-0.1,-0.82,-0.3));
#3633=CARTESIAN_POINT('',(0.,-0.82,-0.3));
#3634=CARTESIAN_POINT('',(0.,-0.82,-0.15));
#3635=CARTESIAN_POINT('',(30.,-0.82,-0.3));
#3636=CARTESIAN_POINT('',(-0.1,-0.82,-0.3));
#3637=CARTESIAN_POINT('',(30.,-0.82,-0.15));
#3638=CARTESIAN_POINT('Origin',(-0.1,-1.05,-0.3));
#3639=CARTESIAN_POINT('',(0.,-1.,-0.3));
#3640=CARTESIAN_POINT('',(0.,-0.525,-0.3));
#3641=CARTESIAN_POINT('',(30.,-1.,-0.3));
#3642=CARTESIAN_POINT('',(-0.05,-1.,-0.3));
#3643=CARTESIAN_POINT('',(30.,-0.525,-0.3));
#3644=CARTESIAN_POINT('Origin',(-0.1,0.3,0.82));
#3645=CARTESIAN_POINT('',(0.,0.3,0.82));
#3646=CARTESIAN_POINT('',(0.,0.3,1.));
#3647=CARTESIAN_POINT('',(0.,0.3,0.41));
#3648=CARTESIAN_POINT('',(30.,0.3,0.82));
#3649=CARTESIAN_POINT('',(-0.1,0.3,0.82));
#3650=CARTESIAN_POINT('',(30.,0.3,1.));
#3651=CARTESIAN_POINT('',(30.,0.3,0.41));
#3652=CARTESIAN_POINT('',(-0.05,0.3,1.));
#3653=CARTESIAN_POINT('Origin',(-0.1,0.55,0.82));
#3654=CARTESIAN_POINT('',(0.,0.55,0.82));
#3655=CARTESIAN_POINT('',(0.,0.275,0.82));
#3656=CARTESIAN_POINT('',(30.,0.55,0.82));
#3657=CARTESIAN_POINT('',(-0.1,0.55,0.82));
#3658=CARTESIAN_POINT('',(30.,0.275,0.82));
#3659=CARTESIAN_POINT('Origin',(-0.1,0.55,0.67));
#3660=CARTESIAN_POINT('',(0.,0.55,0.67));
#3661=CARTESIAN_POINT('',(0.,0.55,0.335));
#3662=CARTESIAN_POINT('',(30.,0.55,0.67));
#3663=CARTESIAN_POINT('',(-0.1,0.55,0.67));
#3664=CARTESIAN_POINT('',(30.,0.55,0.335));
#3665=CARTESIAN_POINT('Origin',(-0.1,0.3,0.42));
#3666=CARTESIAN_POINT('',(0.,0.3,0.42));
#3667=CARTESIAN_POINT('',(6.93889390390723E-18,0.12,0.24));
#3668=CARTESIAN_POINT('',(30.,0.3,0.42));
#3669=CARTESIAN_POINT('',(-0.1,0.3,0.42));
#3670=CARTESIAN_POINT('',(30.,0.12,0.24));
#3671=CARTESIAN_POINT('Origin',(-0.1,-0.3,0.42));
#3672=CARTESIAN_POINT('',(0.,-0.3,0.42));
#3673=CARTESIAN_POINT('',(0.,-0.15,0.42));
#3674=CARTESIAN_POINT('',(30.,-0.3,0.42));
#3675=CARTESIAN_POINT('',(-0.1,-0.3,0.42));
#3676=CARTESIAN_POINT('',(30.,-0.15,0.42));
#3677=CARTESIAN_POINT('Origin',(-0.1,-0.55,0.67));
#3678=CARTESIAN_POINT('',(0.,-0.55,0.67));
#3679=CARTESIAN_POINT('',(6.93889390390723E-18,-0.245,0.365));
#3680=CARTESIAN_POINT('',(30.,-0.55,0.67));
#3681=CARTESIAN_POINT('',(-0.1,-0.55,0.67));
#3682=CARTESIAN_POINT('',(30.,-0.245,0.365));
#3683=CARTESIAN_POINT('Origin',(-0.1,-0.55,0.82));
#3684=CARTESIAN_POINT('',(0.,-0.55,0.82));
#3685=CARTESIAN_POINT('',(0.,-0.55,0.41));
#3686=CARTESIAN_POINT('',(30.,-0.55,0.82));
#3687=CARTESIAN_POINT('',(-0.1,-0.55,0.82));
#3688=CARTESIAN_POINT('',(30.,-0.55,0.41));
#3689=CARTESIAN_POINT('Origin',(-0.1,-0.3,0.82));
#3690=CARTESIAN_POINT('',(0.,-0.3,0.82));
#3691=CARTESIAN_POINT('',(0.,-0.15,0.82));
#3692=CARTESIAN_POINT('',(30.,-0.3,0.82));
#3693=CARTESIAN_POINT('',(-0.1,-0.3,0.82));
#3694=CARTESIAN_POINT('',(30.,-0.15,0.82));
#3695=CARTESIAN_POINT('Origin',(-0.1,-0.3,1.05));
#3696=CARTESIAN_POINT('',(0.,-0.3,1.));
#3697=CARTESIAN_POINT('',(0.,-0.3,0.525));
#3698=CARTESIAN_POINT('',(30.,-0.3,1.));
#3699=CARTESIAN_POINT('',(-0.05,-0.3,1.));
#3700=CARTESIAN_POINT('',(30.,-0.3,0.525));
#3701=CARTESIAN_POINT('Origin',(-0.1,0.,0.));
#3702=CARTESIAN_POINT('',(0.,-2.57175827820944E-17,0.21));
#3703=CARTESIAN_POINT('Origin',(0.,0.,0.));
#3704=CARTESIAN_POINT('',(30.,2.57175827820944E-17,0.21));
#3705=CARTESIAN_POINT('',(-0.1,-2.57175827820944E-17,0.21));
#3706=CARTESIAN_POINT('Origin',(30.,0.,0.));
#3707=CARTESIAN_POINT('Origin',(0.,1.,-1.));
#3708=CARTESIAN_POINT('',(0.,1.,1.));
#3709=CARTESIAN_POINT('',(0.,1.,-1.));
#3710=CARTESIAN_POINT('',(30.,1.,1.));
#3711=CARTESIAN_POINT('',(0.,1.,1.));
#3712=CARTESIAN_POINT('',(30.,1.,-1.));
#3713=CARTESIAN_POINT('Origin',(0.,1.,-1.));
#3714=CARTESIAN_POINT('',(30.,1.,-1.));
#3715=CARTESIAN_POINT('',(30.,1.,-1.));
#3716=CARTESIAN_POINT('',(0.,1.,-1.));
#3717=CARTESIAN_POINT('',(0.,1.,-1.));
#3718=CARTESIAN_POINT('',(0.,1.,-1.));
#3719=CARTESIAN_POINT('Origin',(0.,-1.,-1.));
#3720=CARTESIAN_POINT('',(0.,-1.,-1.));
#3721=CARTESIAN_POINT('',(30.,-1.,-1.));
#3722=CARTESIAN_POINT('Origin',(0.,-1.,-1.));
#3723=CARTESIAN_POINT('',(30.,-1.,-1.));
#3724=CARTESIAN_POINT('',(30.,-1.,-1.));
#3725=CARTESIAN_POINT('',(0.,-1.,-1.));
#3726=CARTESIAN_POINT('',(0.,-1.,-1.));
#3727=CARTESIAN_POINT('',(0.,-1.,-1.));
#3728=CARTESIAN_POINT('Origin',(0.,-1.,1.));
#3729=CARTESIAN_POINT('',(0.,-1.,1.));
#3730=CARTESIAN_POINT('',(30.,-1.,1.));
#3731=CARTESIAN_POINT('Origin',(0.,-1.,1.));
#3732=CARTESIAN_POINT('',(30.,-1.,1.));
#3733=CARTESIAN_POINT('',(30.,-1.,1.));
#3734=CARTESIAN_POINT('',(0.,-1.,1.));
#3735=CARTESIAN_POINT('',(0.,-1.,1.));
#3736=CARTESIAN_POINT('',(0.,-1.,1.));
#3737=CARTESIAN_POINT('Origin',(0.,1.,1.));
#3738=CARTESIAN_POINT('',(0.,1.,1.));
#3739=CARTESIAN_POINT('',(30.,1.,1.));
#3740=CARTESIAN_POINT('Origin',(0.,1.,1.));
#3741=CARTESIAN_POINT('',(30.,1.,1.));
#3742=CARTESIAN_POINT('',(0.,1.,1.));
#3743=CARTESIAN_POINT('Origin',(30.,0.,0.));
#3744=CARTESIAN_POINT('Origin',(0.,0.,0.));
#3759=UNCERTAINTY_MEASURE_WITH_UNIT(LENGTH_MEASURE(0.001),#3774,
'DISTANCE_ACCURACY_VALUE',
'Maximum model space distance between geometric entities at asserted c
onnectivities');
#3760=UNCERTAINTY_MEASURE_WITH_UNIT(LENGTH_MEASURE(0.001),#3774,
'DISTANCE_ACCURACY_VALUE',
'Maximum model space distance between geometric entities at asserted c
onnectivities');
#3772=(
GEOMETRIC_REPRESENTATION_CONTEXT(3)
GLOBAL_UNCERTAINTY_ASSIGNED_CONTEXT((#3759))
GLOBAL_UNIT_ASSIGNED_CONTEXT((#3774,#3776,#3777))
REPRESENTATION_CONTEXT('','3D')
);
#3773=(
GEOMETRIC_REPRESENTATION_CONTEXT(3)
GLOBAL_UNCERTAINTY_ASSIGNED_CONTEXT((#3760))
GLOBAL_UNIT_ASSIGNED_CONTEXT((#3774,#3776,#3777))
REPRESENTATION_CONTEXT('','3D')
);
#3774=(
LENGTH_UNIT()
NAMED_UNIT(*)
SI_UNIT(.CENTI.,.METRE.)
);
#3776=(
NAMED_UNIT(*)
PLANE_ANGLE_UNIT()
SI_UNIT($,.RADIAN.)
);
#3777=(
NAMED_UNIT(*)
SI_UNIT($,.STERADIAN.)
SOLID_ANGLE_UNIT()
);
#3789=SHAPE_DEFINITION_REPRESENTATION(#3809,#3824);
#3809=PRODUCT_DEFINITION_SHAPE('',$,#3837);
#3824=SHAPE_REPRESENTATION('',(#2449),#3772);
#3825=PRODUCT_DEFINITION_CONTEXT('part definition',#3863,'design');
#3837=PRODUCT_DEFINITION('Slotted Extrusion - 20 x 20 x 300 mm',
'Slotted Extrusion - 20 x 20 x 300 mm',#3849,#3825);
#3849=PRODUCT_DEFINITION_FORMATION('',$,#3876);
#3863=APPLICATION_CONTEXT(
'Core Data for Automotive Mechanical Design Process');
#3864=PRODUCT_CONTEXT('part definition',#3863,'mechanical');
#3876=PRODUCT('Slotted Extrusion - 20 x 20 x 300 mm',
'Slotted Extrusion - 20 x 20 x 300 mm',
'Slotted Extrusion - 20 x 20 x 300 mm',(#3864));
#3954=COLOUR_RGB('Off White',0.89,0.88,0.83);
#3955=FILL_AREA_STYLE_COLOUR('',#3954);
#3956=FILL_AREA_STYLE('',(#3955));
#3957=SURFACE_STYLE_FILL_AREA(#3956);
#3958=SURFACE_SIDE_STYLE('',(#3957));
#3959=SURFACE_STYLE_USAGE(.BOTH.,#3958);
#3960=PRESENTATION_STYLE_ASSIGNMENT((#3959));
ENDSEC;
END-ISO-10303-21;
